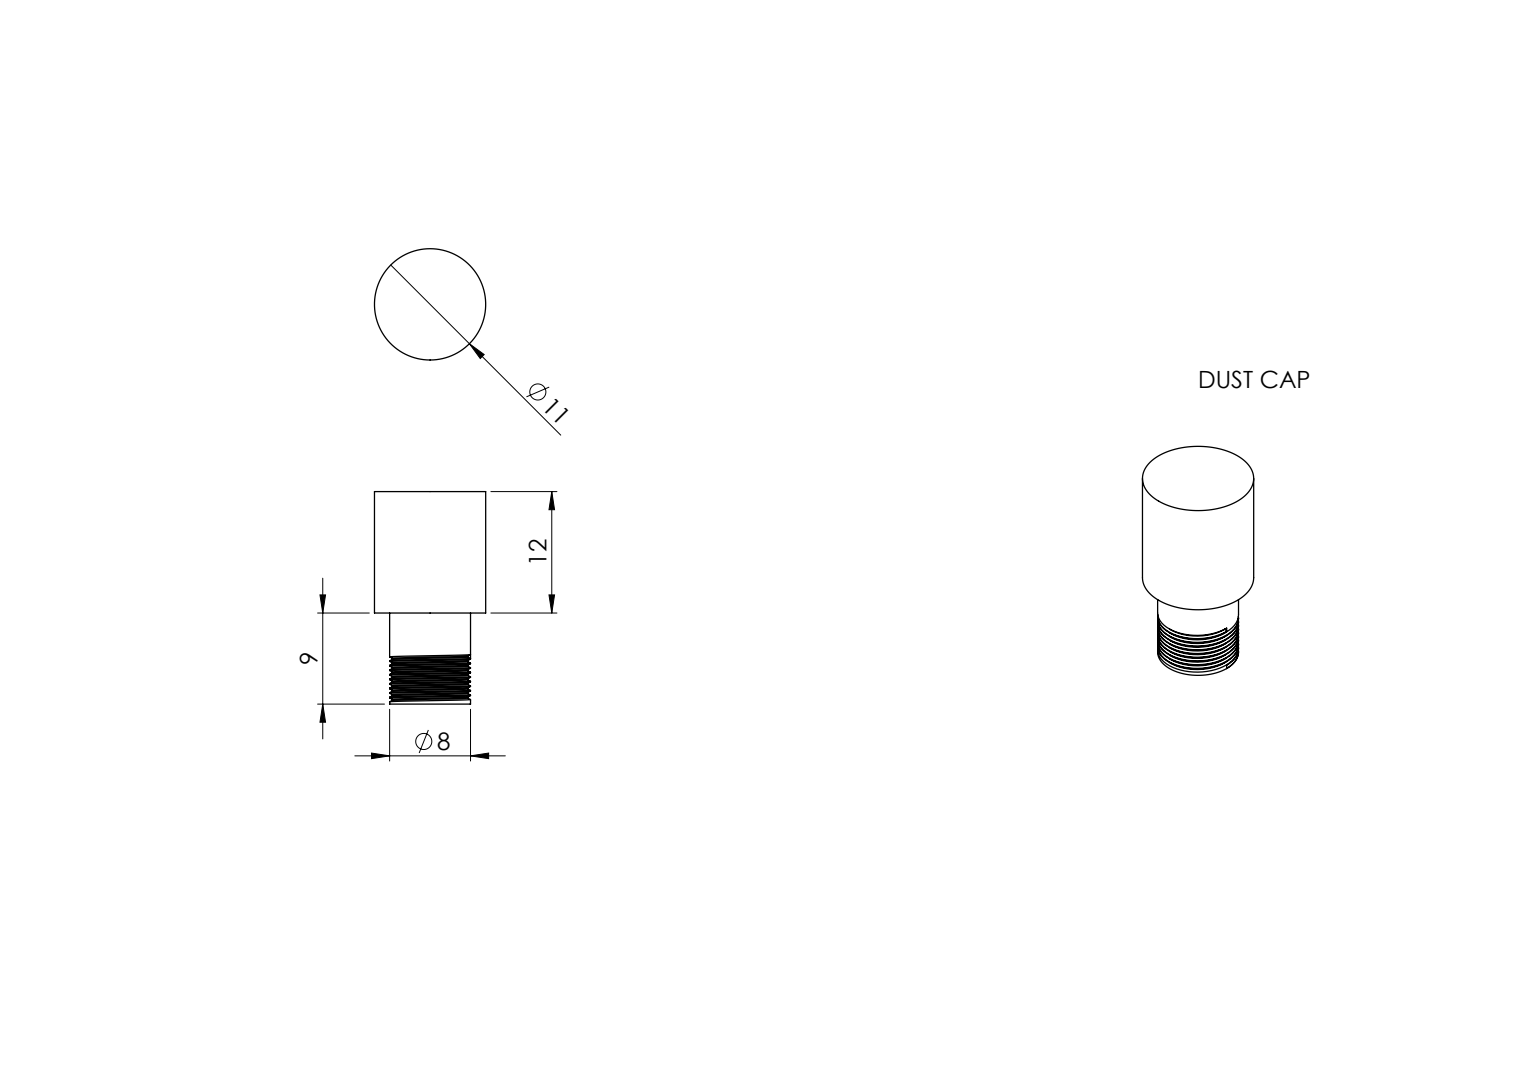
ISO-10303-21;
HEADER;
FILE_DESCRIPTION (('STEP AP214'),
    '1' );
FILE_NAME ('dust cap.step',
    '2026-10-26T12:50:16',
    ( '' ),
    ( '' ),
    'SwSTEP 2.0',
    'SolidWorks 2026',
    '' );
FILE_SCHEMA (( 'AUTOMOTIVE_DESIGN' ));
ENDSEC;

DATA;
#26=CARTESIAN_POINT ( 'NONE',  ( 3.959305671612554781E-15, 40.00000000000000000, 12.99999999999999289 ) ) ;
#57=CARTESIAN_POINT ( 'NONE',  ( 1.071796769724492338, 29.80134618820330417, 12.99999999999999467 ) ) ;
#68=CARTESIAN_POINT ( 'NONE',  ( -3.756430356249996994, 26.26562499938548711, 8.999999999999992895 ) ) ;
#90=CARTESIAN_POINT ( 'NONE',  ( 4.000000000000003553, 27.19374999877096855, 8.999999999999992895 ) ) ;
#94=CARTESIAN_POINT ( 'NONE',  ( 3.756430356250002323, 29.26562499938548356, 11.16877607737301403 ) ) ;
#120=CARTESIAN_POINT ( 'NONE',  ( 3.756430356250002323, 27.01562499938548356, 11.16877607737301226 ) ) ;
#140=VECTOR ( 'NONE', #15561, 1000.000000000000000 ) ;
#148=CARTESIAN_POINT ( 'NONE',  ( -3.756430356249997438, 26.30312499938548854, 11.16877607737301048 ) ) ;
#181=( BOUNDED_CURVE ( )  B_SPLINE_CURVE ( 2, ( #6217, #22433, #20464, #14467, #6482, #24270, #342, #4511, #8455 ),
 .UNSPECIFIED., .F., .T. ) 
 B_SPLINE_CURVE_WITH_KNOTS ( ( 3, 2, 2, 2, 3 ),
 ( 0.02500000000000000139, 0.03333333333333333287, 0.05000000000000000278, 0.06666666666666666574, 0.07500000000000001110 ),
 .UNSPECIFIED. ) 
 CURVE ( )  GEOMETRIC_REPRESENTATION_ITEM ( )  RATIONAL_B_SPLINE_CURVE ( ( 0.9330127018922194093, 0.9330127018922194093, 1.000000000000000000, 0.8660254037844387076, 1.000000000000000000, 0.8660254037844387076, 1.000000000000000000, 0.9330127018922191873, 0.9330127018922192983 ) ) 
 REPRESENTATION_ITEM ( '' )  );
#195=CARTESIAN_POINT ( 'NONE',  ( -3.756430356249997882, 27.20312499938548001, 11.16877607737301226 ) ) ;
#214=CARTESIAN_POINT ( 'NONE',  ( -1.999999999999995781, 28.69374999877096855, 5.535898384862237620 ) ) ;
#218=CARTESIAN_POINT ( 'NONE',  ( 3.756430356250002323, 27.46562499938548640, 11.16877607737301403 ) ) ;
#220=CARTESIAN_POINT ( 'NONE',  ( -3.999999999999997335, 27.90624999877097068, 11.30940107675849404 ) ) ;
#221=ORIENTED_EDGE ( 'NONE', *, *, #3705, .F. ) ;
#222=ORIENTED_EDGE ( 'NONE', *, *, #22140, .F. ) ;
#243=CARTESIAN_POINT ( 'NONE',  ( 3.756430356250003655, 29.75312499938548783, 8.999999999999992895 ) ) ;
#262=CARTESIAN_POINT ( 'NONE',  ( -3.999999999999997335, 27.00624999877096855, 11.30940107675849404 ) ) ;
#263=CARTESIAN_POINT ( 'NONE',  ( 3.834746474454188013E-15, 26.40624999877096357, 4.999999999999992006 ) ) ;
#269=LINE ( 'NONE', #15826, #13033 ) ;
#270=ADVANCED_FACE ( 'NONE', ( #14589 ), #20734, .T. ) ;
#271=CARTESIAN_POINT ( 'NONE',  ( -3.756430356249996994, 25.81562499938548427, 8.999999999999992895 ) ) ;
#287=ORIENTED_EDGE ( 'NONE', *, *, #24315, .F. ) ;
#291=CARTESIAN_POINT ( 'NONE',  ( 2.620986760973688460E-15, 29.38749999999999929, 13.61880215351699874 ) ) ;
#300=EDGE_CURVE ( 'NONE', #5668, #20971, #6231, .T. ) ;
#318=CARTESIAN_POINT ( 'NONE',  ( 2.672651547586948120E-15, 28.17812499938548143, 13.33755215474602984 ) ) ;
#334=CARTESIAN_POINT ( 'NONE',  ( -1.999999999999998224, 26.59374999877096712, 12.46410161513774639 ) ) ;
#342=CARTESIAN_POINT ( 'NONE',  ( -1.999999999999998224, 25.69374999877097210, 12.46410161513774639 ) ) ;
#367=CARTESIAN_POINT ( 'NONE',  ( -1.878215178124995832, 26.19062499938548427, 5.746835883940462963 ) ) ;
#378=( BOUNDED_SURFACE ( )  B_SPLINE_SURFACE ( 1, 2, ( 
 ( #13327, #4838, #19341, #20924, #22880, #1434, #9406, #21174, #3135, #17002, #12814, #4962, #7189, #20786, #15037, #25350, #2867, #13081, #11220, #6925, #23017, #1299, #25102, #18831, #16884, #24849, #12943, #3008, #5102, #19080, #21056, #1160, #9139, #17891, #17645, #21682, #17504, #1943, #3518, #25864, #15939, #3767, #9522, #1554, #21822, #11746, #11489, #120, #9906, #11875, #9662, #25615, #7952, #19726, #15556, #25482, #1823, #13976, #7819, #7568, #11990, #23525, #23911, #18034, #23770, #5859, #13843, #1686, #8091, #3904, #15800, #5992, #19842, #7699, #19964, #5609, #21945, #4023, #2068, #10036, #9787, #23392, #17767, #13589, #15680, #5476, #25736, #5725, #13471, #21437, #19462, #21556, #3636, #11608, #19582, #23648, #13706, #4676, #10672, #22594, #20627, #12655, #2710, #10549, #12262, #18662, #18165, #2327, #20231, #18548, #10286, #12513, #6115, #4291, #16325, #4150, #2586, #22063, #16070, #16187, #243 ),
 ( #505, #8213, #8475, #749, #24153, #16461, #2208, #24033, #14098, #10408, #6244, #16579, #12128, #20104, #10167, #6623, #24538, #22329, #24294, #4411, #14234, #22204, #6379, #18279, #24423, #2447, #6500, #14485, #367, #18407, #8337, #14369, #12385, #20489, #14613, #22452, #20351, #4533, #630, #8597, #3101, #21023, #1013, #4808, #24934, #3347, #8990, #10801, #2833, #13173, #6764, #9102, #21142, #19168, #11184, #25065, #3214, #24678, #11067, #13290, #19045, #17092, #881, #7284, #12783, #20755, #14750, #16967, #18793, #22728, #8864, #1261, #21266, #1128, #16850, #25206, #24814, #7153, #4924, #14875, #23112, #9246, #15143, #15261, #17234, #15000, #12908, #19305, #23229, #5312, #6892, #5194, #11323, #8718, #16705, #2972, #13044, #22850, #20884, #10939, #18930, #7013, #22979, #5065, #21911, #5441, #15767, #13673, #23733, #21644, #9623, #15523, #23491, #23352, #3727, #7401, #9756, #17735, #19429, #3604, #1402 ) ),
 .UNSPECIFIED., .F., .F., .F. ) 
 B_SPLINE_SURFACE_WITH_KNOTS ( ( 2, 2 ),
 ( 3, 2, 2, 2, 2, 2, 2, 2, 2, 2, 2, 2, 2, 2, 2, 2, 2, 2, 2, 2, 2, 2, 2, 2, 2, 2, 2, 2, 2, 2, 2, 2, 2, 2, 2, 2, 2, 2, 2, 2, 2, 2, 2, 2, 2, 2, 2, 2, 2, 2, 2, 2, 2, 2, 2, 2, 2, 2, 2, 2, 3 ),
 ( 0.000000000000000000, 1.000000000000000000 ),
 ( 0.000000000000000000, 0.01666666666666666644, 0.03333333333333333287, 0.05000000000000000278, 0.06666666666666666574, 0.08333333333333332871, 0.1000000000000000056, 0.1166666666666666685, 0.1333333333333333315, 0.1499999999999999944, 0.1666666666666666574, 0.1833333333333333204, 0.2000000000000000111, 0.2166666666666666741, 0.2333333333333333370, 0.2500000000000000000, 0.2666666666666666630, 0.2833333333333333259, 0.2999999999999999889, 0.3166666666666666519, 0.3333333333333333148, 0.3499999999999999778, 0.3666666666666666408, 0.3833333333333333592, 0.4000000000000000222, 0.4166666666666666852, 0.4333333333333333481, 0.4500000000000000111, 0.4666666666666666741, 0.4833333333333333370, 0.5000000000000000000, 0.5166666666666667185, 0.5333333333333333259, 0.5500000000000000444, 0.5666666666666666519, 0.5833333333333333703, 0.5999999999999999778, 0.6166666666666666963, 0.6333333333333333037, 0.6500000000000000222, 0.6666666666666666297, 0.6833333333333333481, 0.6999999999999999556, 0.7166666666666666741, 0.7333333333333332815, 0.7500000000000000000, 0.7666666666666667185, 0.7833333333333333259, 0.8000000000000000444, 0.8166666666666666519, 0.8333333333333333703, 0.8499999999999999778, 0.8666666666666666963, 0.8833333333333333037, 0.9000000000000000222, 0.9166666666666666297, 0.9333333333333333481, 0.9499999999999999556, 0.9666666666666666741, 0.9833333333333332815, 1.000000000000000000 ),
 .UNSPECIFIED. ) 
 GEOMETRIC_REPRESENTATION_ITEM ( )  RATIONAL_B_SPLINE_SURFACE ( (
 ( 1.000000000000000000, 0.8660254037844387076, 1.000000000000000000, 0.8660254037844387076, 1.000000000000000000, 0.8660254037844387076, 1.000000000000000000, 0.8660254037844387076, 1.000000000000000000, 0.8660254037844387076, 1.000000000000000000, 0.8660254037844387076, 1.000000000000000000, 0.8660254037844387076, 1.000000000000000000, 0.8660254037844387076, 1.000000000000000000, 0.8660254037844387076, 1.000000000000000000, 0.8660254037844387076, 1.000000000000000000, 0.8660254037844387076, 1.000000000000000000, 0.8660254037844387076, 1.000000000000000000, 0.8660254037844387076, 1.000000000000000000, 0.8660254037844387076, 1.000000000000000000, 0.8660254037844387076, 1.000000000000000000, 0.8660254037844387076, 1.000000000000000000, 0.8660254037844387076, 1.000000000000000000, 0.8660254037844387076, 1.000000000000000000, 0.8660254037844387076, 1.000000000000000000, 0.8660254037844387076, 1.000000000000000000, 0.8660254037844387076, 1.000000000000000000, 0.8660254037844387076, 1.000000000000000000, 0.8660254037844387076, 1.000000000000000000, 0.8660254037844387076, 1.000000000000000000, 0.8660254037844387076, 1.000000000000000000, 0.8660254037844387076, 1.000000000000000000, 0.8660254037844387076, 1.000000000000000000, 0.8660254037844387076, 1.000000000000000000, 0.8660254037844387076, 1.000000000000000000, 0.8660254037844387076, 1.000000000000000000, 0.8660254037844387076, 1.000000000000000000, 0.8660254037844387076, 1.000000000000000000, 0.8660254037844387076, 1.000000000000000000, 0.8660254037844387076, 1.000000000000000000, 0.8660254037844387076, 1.000000000000000000, 0.8660254037844387076, 1.000000000000000000, 0.8660254037844387076, 1.000000000000000000, 0.8660254037844387076, 1.000000000000000000, 0.8660254037844387076, 1.000000000000000000, 0.8660254037844387076, 1.000000000000000000, 0.8660254037844387076, 1.000000000000000000, 0.8660254037844387076, 1.000000000000000000, 0.8660254037844387076, 1.000000000000000000, 0.8660254037844387076, 1.000000000000000000, 0.8660254037844387076, 1.000000000000000000, 0.8660254037844387076, 1.000000000000000000, 0.8660254037844387076, 1.000000000000000000, 0.8660254037844387076, 1.000000000000000000, 0.8660254037844387076, 1.000000000000000000, 0.8660254037844387076, 1.000000000000000000, 0.8660254037844387076, 1.000000000000000000, 0.8660254037844387076, 1.000000000000000000, 0.8660254037844387076, 1.000000000000000000, 0.8660254037844387076, 1.000000000000000000, 0.8660254037844387076, 1.000000000000000000, 0.8660254037844387076, 1.000000000000000000, 0.8660254037844387076, 1.000000000000000000, 0.8660254037844387076, 1.000000000000000000, 0.8660254037844387076, 1.000000000000000000, 0.8660254037844387076, 1.000000000000000000),
 ( 1.000000000000000000, 0.8660254037844387076, 1.000000000000000000, 0.8660254037844387076, 1.000000000000000000, 0.8660254037844387076, 1.000000000000000000, 0.8660254037844387076, 1.000000000000000000, 0.8660254037844387076, 1.000000000000000000, 0.8660254037844387076, 1.000000000000000000, 0.8660254037844387076, 1.000000000000000000, 0.8660254037844387076, 1.000000000000000000, 0.8660254037844387076, 1.000000000000000000, 0.8660254037844387076, 1.000000000000000000, 0.8660254037844387076, 1.000000000000000000, 0.8660254037844387076, 1.000000000000000000, 0.8660254037844387076, 1.000000000000000000, 0.8660254037844387076, 1.000000000000000000, 0.8660254037844387076, 1.000000000000000000, 0.8660254037844387076, 1.000000000000000000, 0.8660254037844387076, 1.000000000000000000, 0.8660254037844387076, 1.000000000000000000, 0.8660254037844387076, 1.000000000000000000, 0.8660254037844387076, 1.000000000000000000, 0.8660254037844387076, 1.000000000000000000, 0.8660254037844387076, 1.000000000000000000, 0.8660254037844387076, 1.000000000000000000, 0.8660254037844387076, 1.000000000000000000, 0.8660254037844387076, 1.000000000000000000, 0.8660254037844387076, 1.000000000000000000, 0.8660254037844387076, 1.000000000000000000, 0.8660254037844387076, 1.000000000000000000, 0.8660254037844387076, 1.000000000000000000, 0.8660254037844387076, 1.000000000000000000, 0.8660254037844387076, 1.000000000000000000, 0.8660254037844387076, 1.000000000000000000, 0.8660254037844387076, 1.000000000000000000, 0.8660254037844387076, 1.000000000000000000, 0.8660254037844387076, 1.000000000000000000, 0.8660254037844387076, 1.000000000000000000, 0.8660254037844387076, 1.000000000000000000, 0.8660254037844387076, 1.000000000000000000, 0.8660254037844387076, 1.000000000000000000, 0.8660254037844387076, 1.000000000000000000, 0.8660254037844387076, 1.000000000000000000, 0.8660254037844387076, 1.000000000000000000, 0.8660254037844387076, 1.000000000000000000, 0.8660254037844387076, 1.000000000000000000, 0.8660254037844387076, 1.000000000000000000, 0.8660254037844387076, 1.000000000000000000, 0.8660254037844387076, 1.000000000000000000, 0.8660254037844387076, 1.000000000000000000, 0.8660254037844387076, 1.000000000000000000, 0.8660254037844387076, 1.000000000000000000, 0.8660254037844387076, 1.000000000000000000, 0.8660254037844387076, 1.000000000000000000, 0.8660254037844387076, 1.000000000000000000, 0.8660254037844387076, 1.000000000000000000, 0.8660254037844387076, 1.000000000000000000, 0.8660254037844387076, 1.000000000000000000, 0.8660254037844387076, 1.000000000000000000, 0.8660254037844387076, 1.000000000000000000, 0.8660254037844387076, 1.000000000000000000, 0.8660254037844387076, 1.000000000000000000) ) ) 
 REPRESENTATION_ITEM ( '' )  SURFACE ( )  );
#381=EDGE_LOOP ( 'NONE', ( #3819, #17426, #15116, #9054 ) ) ;
#397=CARTESIAN_POINT ( 'NONE',  ( -3.756430356249996105, 25.77812499938548285, 6.831223922626973533 ) ) ;
#408=VERTEX_POINT ( 'NONE', #21244 ) ;
#457=CARTESIAN_POINT ( 'NONE',  ( 2.672651547586948120E-15, 27.27812499938548285, 13.33755215474602984 ) ) ;
#473=CARTESIAN_POINT ( 'NONE',  ( 3.369928719974892281E-15, 25.11250000000000426, 4.999999999999992006 ) ) ;
#477=CARTESIAN_POINT ( 'NONE',  ( -3.756430356249995661, 25.44062499938548427, 6.831223922626973533 ) ) ;
#481=ORIENTED_EDGE ( 'NONE', *, *, #22170, .T. ) ;
#505=CARTESIAN_POINT ( 'NONE',  ( 3.756430356250003655, 25.14062499938548356, 8.999999999999992895 ) ) ;
#535=CARTESIAN_POINT ( 'NONE',  ( -1.878215178124998497, 26.34062499938548285, 12.25316411605951927 ) ) ;
#581=CARTESIAN_POINT ( 'NONE',  ( 1.071796769724494336, 25.09240381056766367, 4.999999999999992895 ) ) ;
#591=CARTESIAN_POINT ( 'NONE',  ( -1.878215178124995832, 27.54062499938548214, 5.746835883940462963 ) ) ;
#597=CARTESIAN_POINT ( 'NONE',  ( 3.369928719974892281E-15, 25.11250000000000426, 4.999999999999992006 ) ) ;
#607=CARTESIAN_POINT ( 'NONE',  ( 3.735045420075836212E-15, 26.26562499938548356, 4.662447845253954171 ) ) ;
#613=( BOUNDED_CURVE ( )  B_SPLINE_CURVE ( 2, ( #5584, #19696, #5450, #11464, #9881 ),
 .UNSPECIFIED., .F., .F. ) 
 B_SPLINE_CURVE_WITH_KNOTS ( ( 3, 2, 3 ),
 ( 0.9749999999999999778, 0.9833333333333332815, 1.000000000000000000 ),
 .UNSPECIFIED. ) 
 CURVE ( )  GEOMETRIC_REPRESENTATION_ITEM ( )  RATIONAL_B_SPLINE_CURVE ( ( 0.9330127018922194093, 0.9330127018922194093, 1.000000000000000000, 0.8660254037844387076, 1.000000000000000000 ) ) 
 REPRESENTATION_ITEM ( '' )  );
#630=CARTESIAN_POINT ( 'NONE',  ( 1.878215178125004048, 26.56562499938548427, 5.746835883940462963 ) ) ;
#632=EDGE_LOOP ( 'NONE', ( #6319, #11612, #8419, #5612 ) ) ;
#657=CARTESIAN_POINT ( 'NONE',  ( 3.756430356250003211, 28.32812499938548356, 6.831223922626973533 ) ) ;
#667=DIRECTION ( 'NONE',  ( 0.000000000000000000, -1.000000000000000000, 0.000000000000000000 ) ) ;
#671=EDGE_LOOP ( 'NONE', ( #19623, #22738 ) ) ;
#683=DIRECTION ( 'NONE',  ( -0.000000000000000000, -1.000000000000000000, -0.000000000000000000 ) ) ;
#706=CARTESIAN_POINT ( 'NONE',  ( 1.071796769724494558, 28.63615380933863364, 4.999999999999992895 ) ) ;
#708=CARTESIAN_POINT ( 'NONE',  ( -3.756430356249996994, 28.51562499938548356, 8.999999999999992895 ) ) ;
#714=EDGE_CURVE ( 'NONE', #10206, #12794, #12708, .T. ) ;
#721=CARTESIAN_POINT ( 'NONE',  ( -1.057460391440397258E-14, 28.71250000000000213, 4.999999999999992006 ) ) ;
#723=CARTESIAN_POINT ( 'NONE',  ( 3.756430356250003655, 26.15312499938548640, 8.999999999999992895 ) ) ;
#728=CARTESIAN_POINT ( 'NONE',  ( 3.756430356250003655, 29.75312499938548783, 8.999999999999992895 ) ) ;
#729=DIRECTION ( 'NONE',  ( 0.000000000000000000, 0.000000000000000000, -1.000000000000000000 ) ) ;
#749=CARTESIAN_POINT ( 'NONE',  ( 3.735045420075836212E-15, 25.25312499938548783, 4.662447845253954171 ) ) ;
#775=CARTESIAN_POINT ( 'NONE',  ( -3.756430356249996994, 29.41562499938548569, 8.999999999999992895 ) ) ;
#803=CARTESIAN_POINT ( 'NONE',  ( 1.859271017917182139E-15, 28.48749999999999716, 12.99999999999999289 ) ) ;
#820=AXIS2_PLACEMENT_3D ( 'NONE', #8589, #18784, #24666 ) ;
#830=ORIENTED_EDGE ( 'NONE', *, *, #3925, .F. ) ;
#832=CARTESIAN_POINT ( 'NONE',  ( 1.878215178125000939, 29.11562499938548498, 12.25316411605952283 ) ) ;
#841=EDGE_CURVE ( 'NONE', #11726, #2271, #16535, .T. ) ;
#851=CARTESIAN_POINT ( 'NONE',  ( -3.999999999999996003, 29.18124999877096926, 6.690598923241487306 ) ) ;
#881=CARTESIAN_POINT ( 'NONE',  ( 1.878215178125004048, 27.46562499938548640, 5.746835883940462963 ) ) ;
#897=ORIENTED_EDGE ( 'NONE', *, *, #8841, .F. ) ;
#910=( BOUNDED_CURVE ( )  B_SPLINE_CURVE ( 2, ( #13594, #7704, #19208, #23776, #5349, #9288, #7824, #17391, #1829 ),
 .UNSPECIFIED., .F., .F. ) 
 B_SPLINE_CURVE_WITH_KNOTS ( ( 3, 2, 2, 2, 3 ),
 ( 0.4750000000000000333, 0.4833333333333333370, 0.5000000000000000000, 0.5166666666666667185, 0.5250000000000000222 ),
 .UNSPECIFIED. ) 
 CURVE ( )  GEOMETRIC_REPRESENTATION_ITEM ( )  RATIONAL_B_SPLINE_CURVE ( ( 0.9330127018922194093, 0.9330127018922196314, 1.000000000000000000, 0.8660254037844387076, 1.000000000000000000, 0.8660254037844387076, 1.000000000000000000, 0.9330127018922194093, 0.9330127018922194093 ) ) 
 REPRESENTATION_ITEM ( '' )  );
#914=CARTESIAN_POINT ( 'NONE',  ( 3.756430356250002323, 29.60312499938548569, 11.16877607737301403 ) ) ;
#966=ORIENTED_EDGE ( 'NONE', *, *, #11818, .F. ) ;
#971=CARTESIAN_POINT ( 'NONE',  ( -1.878215178124998497, 29.04062499938548569, 12.25316411605951927 ) ) ;
#986=CARTESIAN_POINT ( 'NONE',  ( -1.999999999999995781, 29.14374999877096784, 5.535898384862237620 ) ) ;
#1005=ADVANCED_FACE ( 'NONE', ( #19741 ), #11764, .T. ) ;
#1013=CARTESIAN_POINT ( 'NONE',  ( -3.756430356249996994, 26.71562499938548285, 8.999999999999992895 ) ) ;
#1042=CARTESIAN_POINT ( 'NONE',  ( 1.878215178125004048, 29.26562499938548356, 5.746835883940462963 ) ) ;
#1044=LINE ( 'NONE', #17127, #12204 ) ;
#1048=CARTESIAN_POINT ( 'NONE',  ( 3.834746474454188013E-15, 27.75624999877096855, 4.999999999999992006 ) ) ;
#1068=EDGE_CURVE ( 'NONE', #1940, #9674, #15367, .T. ) ;
#1085=ORIENTED_EDGE ( 'NONE', *, *, #12027, .F. ) ;
#1089=CARTESIAN_POINT ( 'NONE',  ( 4.000000000000003553, 25.00000000000000000, 8.999999999999992895 ) ) ;
#1104=CARTESIAN_POINT ( 'NONE',  ( 3.756430356250003655, 27.50312499938548427, 8.999999999999992895 ) ) ;
#1110=CARTESIAN_POINT ( 'NONE',  ( 1.071796769724492338, 26.20134618820330275, 12.99999999999999467 ) ) ;
#1128=CARTESIAN_POINT ( 'NONE',  ( 3.756430356250004099, 27.87812499938548427, 6.831223922626973533 ) ) ;
#1135=CARTESIAN_POINT ( 'NONE',  ( -3.999999999999995559, 28.78750000000000142, 6.690598923241487306 ) ) ;
#1140=CARTESIAN_POINT ( 'NONE',  ( 1.878215178125000939, 26.07812499938548356, 12.25316411605952283 ) ) ;
#1154=CARTESIAN_POINT ( 'NONE',  ( 2.672651547586948120E-15, 28.62812499938548783, 13.33755215474603162 ) ) ;
#1160=CARTESIAN_POINT ( 'NONE',  ( -3.756430356249997882, 26.41562499938548569, 11.16877607737301226 ) ) ;
#1161=CARTESIAN_POINT ( 'NONE',  ( 4.000000000000003553, 27.68124999877096926, 6.690598923241489970 ) ) ;
#1168=VERTEX_POINT ( 'NONE', #8701 ) ;
#1172=EDGE_LOOP ( 'NONE', ( #1838, #14310, #24792, #24076 ) ) ;
#1177=DIRECTION ( 'NONE',  ( -0.000000000000000000, -1.000000000000000000, -0.000000000000000000 ) ) ;
#1214=CARTESIAN_POINT ( 'NONE',  ( -1.878215178124998497, 28.59062499938548285, 12.25316411605951927 ) ) ;
#1219=CARTESIAN_POINT ( 'NONE',  ( -3.999999999999996447, 26.57500000000000284, 8.999999999999992895 ) ) ;
#1233=CARTESIAN_POINT ( 'NONE',  ( -3.756430356249996994, 27.27812499938548640, 8.999999999999992895 ) ) ;
#1261=CARTESIAN_POINT ( 'NONE',  ( 3.756430356250002323, 27.80312499938548143, 11.16877607737301226 ) ) ;
#1273=CARTESIAN_POINT ( 'NONE',  ( -3.756430356249997438, 25.96562499938548640, 11.16877607737301048 ) ) ;
#1299=CARTESIAN_POINT ( 'NONE',  ( 2.672651547586948120E-15, 26.04062499938548925, 13.33755215474602984 ) ) ;
#1300=CARTESIAN_POINT ( 'NONE',  ( 2.000000000000003997, 27.71874999877097068, 5.535898384862238508 ) ) ;
#1305=VERTEX_POINT ( 'NONE', #5426 ) ;
#1326=ADVANCED_FACE ( 'NONE', ( #13414 ), #3053, .T. ) ;
#1356=CARTESIAN_POINT ( 'NONE',  ( -3.999999999999997335, 27.96250000000000213, 11.30940107675849404 ) ) ;
#1359=CARTESIAN_POINT ( 'NONE',  ( -3.137519842735244810E-15, 26.46249999999999858, 4.999999999999991118 ) ) ;
#1360=PRODUCT_DEFINITION ( 'UNKNOWN', '', #16061, #7043 ) ;
#1365=EDGE_CURVE ( 'NONE', #21478, #1940, #2376, .T. ) ;
#1376=CARTESIAN_POINT ( 'NONE',  ( 1.878215178125000939, 27.42812499938548498, 12.25316411605952283 ) ) ;
#1395=FACE_OUTER_BOUND ( 'NONE', #2684, .T. ) ;
#1402=CARTESIAN_POINT ( 'NONE',  ( 3.756430356250003655, 29.64062499938548356, 8.999999999999992895 ) ) ;
#1407=CARTESIAN_POINT ( 'NONE',  ( 2.000000000000000888, 25.76874999877096784, 12.46410161513774817 ) ) ;
#1412=CARTESIAN_POINT ( 'NONE',  ( 1.878215178125000939, 26.97812499938548569, 12.25316411605952283 ) ) ;
#1434=CARTESIAN_POINT ( 'NONE',  ( -3.756430356249995661, 25.44062499938548427, 6.831223922626973533 ) ) ;
#1472=ORIENTED_EDGE ( 'NONE', *, *, #300, .F. ) ;
#1477=CARTESIAN_POINT ( 'NONE',  ( 4.000000000000003553, 26.83749999999999503, 6.690598923241489970 ) ) ;
#1478=ORIENTED_EDGE ( 'NONE', *, *, #8035, .F. ) ;
#1480=CARTESIAN_POINT ( 'NONE',  ( 3.752267015613588906E-15, 28.26250000000000284, 4.381197846482986158 ) ) ;
#1481=CARTESIAN_POINT ( 'NONE',  ( 3.469446951953614189E-15, 46.00000000000000000, 8.999999999999992895 ) ) ;
#1482=CARTESIAN_POINT ( 'NONE',  ( -3.999999999999995559, 26.53750000000000142, 6.690598923241487306 ) ) ;
#1497=CARTESIAN_POINT ( 'NONE',  ( -1.878215178124995832, 28.55312499938548498, 5.746835883940462963 ) ) ;
#1506=CARTESIAN_POINT ( 'NONE',  ( 1.878215178125004048, 25.66562499938548569, 5.746835883940462963 ) ) ;
#1525=CARTESIAN_POINT ( 'NONE',  ( -3.999999999999996003, 25.58124999877097139, 6.690598923241487306 ) ) ;
#1527=FACE_OUTER_BOUND ( 'NONE', #671, .T. ) ;
#1529=CARTESIAN_POINT ( 'NONE',  ( 3.756430356250003211, 26.19062499938548783, 6.831223922626973533 ) ) ;
#1531=ORIENTED_EDGE ( 'NONE', *, *, #3720, .T. ) ;
#1554=CARTESIAN_POINT ( 'NONE',  ( -3.756430356249997882, 26.86562499938548498, 11.16877607737301226 ) ) ;
#1559=DIRECTION ( 'NONE',  ( 0.000000000000000000, 1.000000000000000000, 0.000000000000000000 ) ) ;
#1603=CARTESIAN_POINT ( 'NONE',  ( 4.000000000000003553, 26.38750000000000284, 6.690598923241489970 ) ) ;
#1617=AXIS2_PLACEMENT_3D ( 'NONE', #19728, #19843, #5727 ) ;
#1621=CARTESIAN_POINT ( 'NONE',  ( 3.756430356250004099, 27.09062499938548285, 6.831223922626973533 ) ) ;
#1630=CARTESIAN_POINT ( 'NONE',  ( -3.756430356249996994, 25.36562499938548498, 8.999999999999992895 ) ) ;
#1640=CARTESIAN_POINT ( 'NONE',  ( -3.999999999999997335, 27.51250000000000284, 11.30940107675849404 ) ) ;
#1654=CARTESIAN_POINT ( 'NONE',  ( -3.999999999999996447, 26.06874999877096855, 8.999999999999992895 ) ) ;
#1658=CARTESIAN_POINT ( 'NONE',  ( -3.756430356249996105, 26.34062499938548285, 6.831223922626973533 ) ) ;
#1665=VERTEX_POINT ( 'NONE', #2239 ) ;
#1686=CARTESIAN_POINT ( 'NONE',  ( -3.756430356249997882, 27.76562499938549067, 11.16877607737301226 ) ) ;
#1702=ORIENTED_EDGE ( 'NONE', *, *, #22026, .T. ) ;
#1718=FACE_OUTER_BOUND ( 'NONE', #4223, .T. ) ;
#1720=LINE ( 'NONE', #18068, #3840 ) ;
#1734=LINE ( 'NONE', #26, #23734 ) ;
#1741=CIRCLE ( 'NONE', #5077, 5.500000000000000000 ) ;
#1742=ORIENTED_EDGE ( 'NONE', *, *, #11468, .F. ) ;
#1743=CARTESIAN_POINT ( 'NONE',  ( 2.000000000000000888, 27.62500000000000000, 12.46410161513774817 ) ) ;
#1745=VECTOR ( 'NONE', #14065, 1000.000000000000000 ) ;
#1750=( BOUNDED_CURVE ( )  B_SPLINE_CURVE ( 2, ( #23869, #8175, #5954, #17730, #23996, #1640, #19806, #25699, #18130 ),
 .UNSPECIFIED., .F., .F. ) 
 B_SPLINE_CURVE_WITH_KNOTS ( ( 3, 2, 2, 2, 3 ),
 ( 0.5250000000000000222, 0.5333333333333333259, 0.5500000000000000444, 0.5666666666666666519, 0.5750000000000000666 ),
 .UNSPECIFIED. ) 
 CURVE ( )  GEOMETRIC_REPRESENTATION_ITEM ( )  RATIONAL_B_SPLINE_CURVE ( ( 0.9330127018922194093, 0.9330127018922194093, 1.000000000000000000, 0.8660254037844387076, 1.000000000000000000, 0.8660254037844387076, 1.000000000000000000, 0.9330127018922189652, 0.9330127018922194093 ) ) 
 REPRESENTATION_ITEM ( '' )  );
#1752=CYLINDRICAL_SURFACE ( 'NONE', #20479, 4.000000000000000000 ) ;
#1767=CARTESIAN_POINT ( 'NONE',  ( 3.756430356250004099, 29.34062499938548640, 6.831223922626973533 ) ) ;
#1793=CARTESIAN_POINT ( 'NONE',  ( -1.999999999999995781, 25.99374999877096926, 5.535898384862237620 ) ) ;
#1797=CARTESIAN_POINT ( 'NONE',  ( 2.672651547586948120E-15, 27.84062499938548640, 13.33755215474603162 ) ) ;
#1823=CARTESIAN_POINT ( 'NONE',  ( -1.878215178124998497, 27.35312499938548569, 12.25316411605951927 ) ) ;
#1829=CARTESIAN_POINT ( 'NONE',  ( 3.834746474454188013E-15, 27.36250000000000426, 4.999999999999992006 ) ) ;
#1838=ORIENTED_EDGE ( 'NONE', *, *, #4123, .F. ) ;
#1857=CARTESIAN_POINT ( 'NONE',  ( 1.626862140677534194E-14, 27.58750000000000213, 12.99999999999999289 ) ) ;
#1865=( BOUNDED_CURVE ( )  B_SPLINE_CURVE ( 2, ( #8288, #10502, #16271, #24241, #8427, #24382, #6458, #706, #14446 ),
 .UNSPECIFIED., .F., .F. ) 
 B_SPLINE_CURVE_WITH_KNOTS ( ( 3, 2, 2, 2, 3 ),
 ( 0.6750000000000000444, 0.6833333333333333481, 0.6999999999999999556, 0.7166666666666666741, 0.7249999999999999778 ),
 .UNSPECIFIED. ) 
 CURVE ( )  GEOMETRIC_REPRESENTATION_ITEM ( )  RATIONAL_B_SPLINE_CURVE ( ( 0.9330127018922194093, 0.9330127018922198534, 1.000000000000000000, 0.8660254037844387076, 1.000000000000000000, 0.8660254037844387076, 1.000000000000000000, 0.9330127018922194093, 0.9330127018922194093 ) ) 
 REPRESENTATION_ITEM ( '' )  );
#1869=CARTESIAN_POINT ( 'NONE',  ( 3.369928719974892281E-15, 25.50624999877096855, 4.999999999999992006 ) ) ;
#1872=CARTESIAN_POINT ( 'NONE',  ( 4.000000000000003553, 26.80000000000000071, 8.999999999999992895 ) ) ;
#1874=ADVANCED_FACE ( 'NONE', ( #24967 ), #378, .T. ) ;
#1907=EDGE_CURVE ( 'NONE', #10879, #16189, #17053, .T. ) ;
#1918=CARTESIAN_POINT ( 'NONE',  ( -1.999999999999998224, 28.39374999877096784, 12.46410161513774639 ) ) ;
#1922=CARTESIAN_POINT ( 'NONE',  ( 2.672651547586948120E-15, 28.74062499938548854, 13.33755215474603162 ) ) ;
#1940=VERTEX_POINT ( 'NONE', #13557 ) ;
#1943=CARTESIAN_POINT ( 'NONE',  ( 3.756430356250004099, 26.64062499938549067, 6.831223922626973533 ) ) ;
#1949=DIRECTION ( 'NONE',  ( -0.000000000000000000, -1.000000000000000000, -0.000000000000000000 ) ) ;
#1958=ADVANCED_FACE ( 'NONE', ( #21523 ), #11575, .T. ) ;
#1962=SURFACE_SIDE_STYLE ('',( #8501 ) ) ;
#1964=EDGE_CURVE ( 'NONE', #12794, #16109, #10013, .T. ) ;
#1986=CARTESIAN_POINT ( 'NONE',  ( 1.071796769724494336, 25.48615380933863150, 4.999999999999992895 ) ) ;
#1994=CARTESIAN_POINT ( 'NONE',  ( 3.834746474454188013E-15, 26.01249999999999574, 4.999999999999992006 ) ) ;
#2008=CARTESIAN_POINT ( 'NONE',  ( 2.672651547586948120E-15, 29.19062499938548783, 13.33755215474602984 ) ) ;
#2017=CARTESIAN_POINT ( 'NONE',  ( 3.756430356250003655, 26.04062499938548569, 8.999999999999992895 ) ) ;
#2024=CARTESIAN_POINT ( 'NONE',  ( 8.831537335106614961E-15, 27.13750000000000284, 12.99999999999999112 ) ) ;
#2039=CARTESIAN_POINT ( 'NONE',  ( 2.000000000000000888, 27.56874999877096855, 12.46410161513774817 ) ) ;
#2043=CARTESIAN_POINT ( 'NONE',  ( 3.756430356250003211, 27.99062499938548498, 6.831223922626973533 ) ) ;
#2057=AXIS2_PLACEMENT_3D ( 'NONE', #24683, #18412, #24817 ) ;
#2062=CARTESIAN_POINT ( 'NONE',  ( 1.071796769724494558, 25.54240381056766651, 4.999999999999992895 ) ) ;
#2068=CARTESIAN_POINT ( 'NONE',  ( -3.756430356249996994, 28.17812499938548498, 8.999999999999992895 ) ) ;
#2093=( NAMED_UNIT ( * ) SI_UNIT ( $, .STERADIAN. ) SOLID_ANGLE_UNIT ( ) );
#2097=CARTESIAN_POINT ( 'NONE',  ( 3.756430356250003211, 25.17812499938548498, 6.831223922626973533 ) ) ;
#2155=CARTESIAN_POINT ( 'NONE',  ( 1.878215178125004048, 26.56562499938548427, 5.746835883940462963 ) ) ;
#2176=CARTESIAN_POINT ( 'NONE',  ( -3.999999999999996447, 28.31874999877096855, 8.999999999999992895 ) ) ;
#2180=CARTESIAN_POINT ( 'NONE',  ( 1.878215178125000939, 28.32812499938548711, 12.25316411605952283 ) ) ;
#2193=CIRCLE ( 'NONE', #16817, 5.500000000000000000 ) ;
#2208=CARTESIAN_POINT ( 'NONE',  ( -3.756430356249996994, 25.36562499938548498, 8.999999999999992895 ) ) ;
#2209=AXIS2_PLACEMENT_3D ( 'NONE', #23562, #4189, #23679 ) ;
#2234=CARTESIAN_POINT ( 'NONE',  ( -3.756430356249996105, 25.32812499938548356, 6.831223922626973533 ) ) ;
#2239=CARTESIAN_POINT ( 'NONE',  ( 3.834746474454188013E-15, 27.36250000000000071, 4.999999999999992006 ) ) ;
#2255=CARTESIAN_POINT ( 'NONE',  ( 2.620986760973688460E-15, 28.93750000000000000, 13.61880215351699874 ) ) ;
#2271=VERTEX_POINT ( 'NONE', #18756 ) ;
#2283=CARTESIAN_POINT ( 'NONE',  ( -1.878215178124998497, 28.14062499938548356, 12.25316411605951927 ) ) ;
#2300=CARTESIAN_POINT ( 'NONE',  ( 2.000000000000000888, 26.66874999877096641, 12.46410161513774817 ) ) ;
#2309=CARTESIAN_POINT ( 'NONE',  ( 4.000000000000003553, 29.89374999877096784, 8.999999999999992895 ) ) ;
#2327=CARTESIAN_POINT ( 'NONE',  ( 3.756430356250002323, 29.26562499938548356, 11.16877607737301226 ) ) ;
#2338=ORIENTED_EDGE ( 'NONE', *, *, #8279, .F. ) ;
#2345=EDGE_CURVE ( 'NONE', #22108, #19820, #19079, .T. ) ;
#2350=SURFACE_STYLE_USAGE ( .BOTH. , #1962 ) ;
#2354=CARTESIAN_POINT ( 'NONE',  ( -3.756430356249996994, 25.36562499938548498, 8.999999999999992895 ) ) ;
#2376=LINE ( 'NONE', #12040, #17207 ) ;
#2399=ADVANCED_FACE ( 'NONE', ( #5760 ), #19765, .T. ) ;
#2401=CARTESIAN_POINT ( 'NONE',  ( 3.735045420075836212E-15, 27.05312499938548498, 4.662447845253954171 ) ) ;
#2403=FACE_OUTER_BOUND ( 'NONE', #20273, .T. ) ;
#2415=CARTESIAN_POINT ( 'NONE',  ( 2.000000000000000888, 29.81874999877096855, 12.46410161513774817 ) ) ;
#2423=CARTESIAN_POINT ( 'NONE',  ( -1.071796769724487230, 27.77634618820330559, 4.999999999999992006 ) ) ;
#2447=CARTESIAN_POINT ( 'NONE',  ( 3.756430356250004099, 26.07812499938548356, 6.831223922626973533 ) ) ;
#2452=ORIENTED_EDGE ( 'NONE', *, *, #20965, .F. ) ;
#2463=CARTESIAN_POINT ( 'NONE',  ( -3.999999999999995559, 26.93124999877096926, 6.690598923241487306 ) ) ;
#2468=PRESENTATION_STYLE_ASSIGNMENT (( #2350 ) ) ;
#2473=AXIS2_PLACEMENT_3D ( 'NONE', #12395, #8347, #16079 ) ;
#2475=CARTESIAN_POINT ( 'NONE',  ( 3.735045420075836212E-15, 25.25312499938548427, 4.662447845253954171 ) ) ;
#2484=CARTESIAN_POINT ( 'NONE',  ( -1.999999999999998224, 28.00000000000000000, 12.46410161513774639 ) ) ;
#2493=ORIENTED_EDGE ( 'NONE', *, *, #3693, .F. ) ;
#2528=EDGE_LOOP ( 'NONE', ( #6641, #17739, #11163 ) ) ;
#2534=CARTESIAN_POINT ( 'NONE',  ( 1.878215178125000939, 27.31562499938548427, 12.25316411605952283 ) ) ;
#2536=AXIS2_PLACEMENT_3D ( 'NONE', #15735, #21999, #13642 ) ;
#2554=CARTESIAN_POINT ( 'NONE',  ( -3.756430356249997882, 25.96562499938548640, 11.16877607737301226 ) ) ;
#2569=DIRECTION ( 'NONE',  ( -0.000000000000000000, -1.000000000000000000, -0.000000000000000000 ) ) ;
#2586=CARTESIAN_POINT ( 'NONE',  ( -1.878215178124998497, 29.60312499938548569, 12.25316411605951927 ) ) ;
#2599=EDGE_CURVE ( 'NONE', #5942, #4195, #2627, .T. ) ;
#2615=VECTOR ( 'NONE', #13942, 1000.000000000000000 ) ;
#2618=CARTESIAN_POINT ( 'NONE',  ( 3.756430356250003655, 25.14062499938548356, 8.999999999999992895 ) ) ;
#2627=LINE ( 'NONE', #18454, #20438 ) ;
#2640=ORIENTED_EDGE ( 'NONE', *, *, #8385, .T. ) ;
#2671=CARTESIAN_POINT ( 'NONE',  ( 2.000000000000000888, 25.37500000000000000, 12.46410161513774817 ) ) ;
#2684=EDGE_LOOP ( 'NONE', ( #23658, #14103, #22454, #9448 ) ) ;
#2685=CARTESIAN_POINT ( 'NONE',  ( 2.672651547586948120E-15, 26.04062499938548925, 13.33755215474602984 ) ) ;
#2692=EDGE_CURVE ( 'NONE', #22640, #11825, #5350, .T. ) ;
#2701=DIRECTION ( 'NONE',  ( 0.000000000000000000, 0.000000000000000000, -1.000000000000000000 ) ) ;
#2710=CARTESIAN_POINT ( 'NONE',  ( -3.756430356249996994, 29.07812499938548356, 8.999999999999992895 ) ) ;
#2716=CARTESIAN_POINT ( 'NONE',  ( 3.834746474454188013E-15, 25.95624999877096428, 4.999999999999992006 ) ) ;
#2739=CARTESIAN_POINT ( 'NONE',  ( 3.756430356250003655, 28.29062499938548569, 8.999999999999992895 ) ) ;
#2755=ORIENTED_EDGE ( 'NONE', *, *, #2599, .F. ) ;
#2772=EDGE_CURVE ( 'NONE', #2907, #4929, #9413, .T. ) ;
#2789=CARTESIAN_POINT ( 'NONE',  ( -3.756430356249995661, 28.92812499938548143, 6.831223922626973533 ) ) ;
#2790=CARTESIAN_POINT ( 'NONE',  ( -3.999999999999995559, 28.28124999877096712, 6.690598923241487306 ) ) ;
#2806=CARTESIAN_POINT ( 'NONE',  ( 2.672651547586948120E-15, 25.59062499938548640, 13.33755215474602984 ) ) ;
#2833=CARTESIAN_POINT ( 'NONE',  ( 3.756430356250003655, 26.94062499938548427, 8.999999999999992895 ) ) ;
#2845=ADVANCED_FACE ( 'NONE', ( #17653 ), #23918, .T. ) ;
#2862=CARTESIAN_POINT ( 'NONE',  ( -1.878215178124995832, 28.44062499938548427, 5.746835883940462963 ) ) ;
#2867=CARTESIAN_POINT ( 'NONE',  ( -1.878215178124995832, 25.85312499938548569, 5.746835883940462963 ) ) ;
#2896=ADVANCED_FACE ( 'NONE', ( #3775 ), #25623, .T. ) ;
#2907=VERTEX_POINT ( 'NONE', #21951 ) ;
#2924=CARTESIAN_POINT ( 'NONE',  ( -1.999999999999998224, 25.75000000000000355, 12.46410161513774639 ) ) ;
#2925=CARTESIAN_POINT ( 'NONE',  ( 1.071796769724491227, 27.28615380933863577, 4.999999999999989342 ) ) ;
#2931=CARTESIAN_POINT ( 'NONE',  ( -1.071796769724488563, 28.46740381056766722, 12.99999999999999289 ) ) ;
#2942=CARTESIAN_POINT ( 'NONE',  ( -1.999999999999998224, 29.29374999877096997, 12.46410161513774639 ) ) ;
#2972=CARTESIAN_POINT ( 'NONE',  ( 3.756430356250002323, 28.70312499938548356, 11.16877607737301226 ) ) ;
#2987=EDGE_LOOP ( 'NONE', ( #21157, #16477, #16651, #17394 ) ) ;
#3001=CARTESIAN_POINT ( 'NONE',  ( -3.756430356249996105, 28.47812499938548569, 6.831223922626973533 ) ) ;
#3008=CARTESIAN_POINT ( 'NONE',  ( 3.735045420075836212E-15, 26.26562499938548356, 4.662447845253954171 ) ) ;
#3010=CARTESIAN_POINT ( 'NONE',  ( -1.071796769724493448, 29.57634618820329564, 4.999999999999995559 ) ) ;
#3012=LINE ( 'NONE', #19083, #140 ) ;
#3053=( BOUNDED_SURFACE ( )  B_SPLINE_SURFACE ( 1, 2, ( 
 ( #23602, #19669, #5561, #21389, #3589, #13275, #1630, #3469, #11441, #15754, #11307, #23717, #3329, #19413, #1506, #9477, #17455, #25425, #7512, #15506, #23473, #17590, #23987, #4487, #2017, #17978, #11946, #14181, #9985, #19916, #68, #24383, #18503, #18235, #3981, #22407, #16023, #16273, #2155, #12076, #20307, #6460, #24242, #12463, #10358, #12215, #10123, #16539, #20436, #14447, #8041, #2401, #16415, #5944, #12343, #195, #10238, #457, #2534, #10503, #18359, #8428, #4098, #6330, #591, #6070, #8557, #13930, #6191, #22151, #21898, #14053, #18122, #22019, #8168, #20050, #16147, #24108, #4236, #20184, #2283, #318, #8289, #14323, #22287, #4366, #25016, #3057, #10884, #8953, #708, #16927, #1214, #9195, #7105, #14705, #8676, #13129, #19006, #24895, #22806, #2789, #24501, #16657, #971, #14562, #832, #11026, #5153, #6850, #6973, #24624, #10753, #5015, #18884, #6580, #19122, #22543, #4623, #22928, #14953 ),
 ( #1089, #18743, #4883, #18623, #9063, #12606, #17045, #15090, #12856, #10631, #2671, #12997, #20833, #20581, #6710, #23068, #20977, #8809, #16802, #21099, #2924, #22683, #4768, #3177, #11143, #12739, #20710, #24768, #14833, #21605, #11801, #17561, #25536, #7621, #21357, #19776, #15607, #1603, #11660, #23576, #11413, #5773, #11271, #9573, #17697, #19637, #13757, #13518, #1872, #21487, #7361, #19256, #21736, #3562, #3820, #11536, #9715, #19503, #5654, #25157, #5270, #13636, #17431, #17183, #7240, #15219, #23692, #23185, #13248, #3682, #1743, #25666, #7745, #25397, #5391, #13382, #21217, #15728, #3298, #1356, #9333, #17317, #19387, #25280, #15339, #23307, #3441, #1480, #9451, #7484, #15473, #23442, #5532, #23961, #7866, #11919, #20155, #21871, #22375, #9834, #4203, #9955, #10331, #17817, #5911, #2255, #19889, #14149, #24348, #18088, #16117, #13899, #8008, #10087, #25782, #18209, #22115, #291, #8260, #6043, #12181 ) ),
 .UNSPECIFIED., .F., .F., .F. ) 
 B_SPLINE_SURFACE_WITH_KNOTS ( ( 2, 2 ),
 ( 3, 2, 2, 2, 2, 2, 2, 2, 2, 2, 2, 2, 2, 2, 2, 2, 2, 2, 2, 2, 2, 2, 2, 2, 2, 2, 2, 2, 2, 2, 2, 2, 2, 2, 2, 2, 2, 2, 2, 2, 2, 2, 2, 2, 2, 2, 2, 2, 2, 2, 2, 2, 2, 2, 2, 2, 2, 2, 2, 2, 3 ),
 ( 0.000000000000000000, 1.000000000000000000 ),
 ( 0.000000000000000000, 0.01666666666666666644, 0.03333333333333333287, 0.05000000000000000278, 0.06666666666666666574, 0.08333333333333332871, 0.1000000000000000056, 0.1166666666666666685, 0.1333333333333333315, 0.1499999999999999944, 0.1666666666666666574, 0.1833333333333333204, 0.2000000000000000111, 0.2166666666666666741, 0.2333333333333333370, 0.2500000000000000000, 0.2666666666666666630, 0.2833333333333333259, 0.2999999999999999889, 0.3166666666666666519, 0.3333333333333333148, 0.3499999999999999778, 0.3666666666666666408, 0.3833333333333333592, 0.4000000000000000222, 0.4166666666666666852, 0.4333333333333333481, 0.4500000000000000111, 0.4666666666666666741, 0.4833333333333333370, 0.5000000000000000000, 0.5166666666666667185, 0.5333333333333333259, 0.5500000000000000444, 0.5666666666666666519, 0.5833333333333333703, 0.5999999999999999778, 0.6166666666666666963, 0.6333333333333333037, 0.6500000000000000222, 0.6666666666666666297, 0.6833333333333333481, 0.6999999999999999556, 0.7166666666666666741, 0.7333333333333332815, 0.7500000000000000000, 0.7666666666666667185, 0.7833333333333333259, 0.8000000000000000444, 0.8166666666666666519, 0.8333333333333333703, 0.8499999999999999778, 0.8666666666666666963, 0.8833333333333333037, 0.9000000000000000222, 0.9166666666666666297, 0.9333333333333333481, 0.9499999999999999556, 0.9666666666666666741, 0.9833333333333332815, 1.000000000000000000 ),
 .UNSPECIFIED. ) 
 GEOMETRIC_REPRESENTATION_ITEM ( )  RATIONAL_B_SPLINE_SURFACE ( (
 ( 1.000000000000000000, 0.8660254037844387076, 1.000000000000000000, 0.8660254037844387076, 1.000000000000000000, 0.8660254037844387076, 1.000000000000000000, 0.8660254037844387076, 1.000000000000000000, 0.8660254037844387076, 1.000000000000000000, 0.8660254037844387076, 1.000000000000000000, 0.8660254037844387076, 1.000000000000000000, 0.8660254037844387076, 1.000000000000000000, 0.8660254037844387076, 1.000000000000000000, 0.8660254037844387076, 1.000000000000000000, 0.8660254037844387076, 1.000000000000000000, 0.8660254037844387076, 1.000000000000000000, 0.8660254037844387076, 1.000000000000000000, 0.8660254037844387076, 1.000000000000000000, 0.8660254037844387076, 1.000000000000000000, 0.8660254037844387076, 1.000000000000000000, 0.8660254037844387076, 1.000000000000000000, 0.8660254037844387076, 1.000000000000000000, 0.8660254037844387076, 1.000000000000000000, 0.8660254037844387076, 1.000000000000000000, 0.8660254037844387076, 1.000000000000000000, 0.8660254037844387076, 1.000000000000000000, 0.8660254037844387076, 1.000000000000000000, 0.8660254037844387076, 1.000000000000000000, 0.8660254037844387076, 1.000000000000000000, 0.8660254037844387076, 1.000000000000000000, 0.8660254037844387076, 1.000000000000000000, 0.8660254037844387076, 1.000000000000000000, 0.8660254037844387076, 1.000000000000000000, 0.8660254037844387076, 1.000000000000000000, 0.8660254037844387076, 1.000000000000000000, 0.8660254037844387076, 1.000000000000000000, 0.8660254037844387076, 1.000000000000000000, 0.8660254037844387076, 1.000000000000000000, 0.8660254037844387076, 1.000000000000000000, 0.8660254037844387076, 1.000000000000000000, 0.8660254037844387076, 1.000000000000000000, 0.8660254037844387076, 1.000000000000000000, 0.8660254037844387076, 1.000000000000000000, 0.8660254037844387076, 1.000000000000000000, 0.8660254037844387076, 1.000000000000000000, 0.8660254037844387076, 1.000000000000000000, 0.8660254037844387076, 1.000000000000000000, 0.8660254037844387076, 1.000000000000000000, 0.8660254037844387076, 1.000000000000000000, 0.8660254037844387076, 1.000000000000000000, 0.8660254037844387076, 1.000000000000000000, 0.8660254037844387076, 1.000000000000000000, 0.8660254037844387076, 1.000000000000000000, 0.8660254037844387076, 1.000000000000000000, 0.8660254037844387076, 1.000000000000000000, 0.8660254037844387076, 1.000000000000000000, 0.8660254037844387076, 1.000000000000000000, 0.8660254037844387076, 1.000000000000000000, 0.8660254037844387076, 1.000000000000000000, 0.8660254037844387076, 1.000000000000000000, 0.8660254037844387076, 1.000000000000000000, 0.8660254037844387076, 1.000000000000000000, 0.8660254037844387076, 1.000000000000000000, 0.8660254037844387076, 1.000000000000000000),
 ( 1.000000000000000000, 0.8660254037844387076, 1.000000000000000000, 0.8660254037844387076, 1.000000000000000000, 0.8660254037844387076, 1.000000000000000000, 0.8660254037844387076, 1.000000000000000000, 0.8660254037844387076, 1.000000000000000000, 0.8660254037844387076, 1.000000000000000000, 0.8660254037844387076, 1.000000000000000000, 0.8660254037844387076, 1.000000000000000000, 0.8660254037844387076, 1.000000000000000000, 0.8660254037844387076, 1.000000000000000000, 0.8660254037844387076, 1.000000000000000000, 0.8660254037844387076, 1.000000000000000000, 0.8660254037844387076, 1.000000000000000000, 0.8660254037844387076, 1.000000000000000000, 0.8660254037844387076, 1.000000000000000000, 0.8660254037844387076, 1.000000000000000000, 0.8660254037844387076, 1.000000000000000000, 0.8660254037844387076, 1.000000000000000000, 0.8660254037844387076, 1.000000000000000000, 0.8660254037844387076, 1.000000000000000000, 0.8660254037844387076, 1.000000000000000000, 0.8660254037844387076, 1.000000000000000000, 0.8660254037844387076, 1.000000000000000000, 0.8660254037844387076, 1.000000000000000000, 0.8660254037844387076, 1.000000000000000000, 0.8660254037844387076, 1.000000000000000000, 0.8660254037844387076, 1.000000000000000000, 0.8660254037844387076, 1.000000000000000000, 0.8660254037844387076, 1.000000000000000000, 0.8660254037844387076, 1.000000000000000000, 0.8660254037844387076, 1.000000000000000000, 0.8660254037844387076, 1.000000000000000000, 0.8660254037844387076, 1.000000000000000000, 0.8660254037844387076, 1.000000000000000000, 0.8660254037844387076, 1.000000000000000000, 0.8660254037844387076, 1.000000000000000000, 0.8660254037844387076, 1.000000000000000000, 0.8660254037844387076, 1.000000000000000000, 0.8660254037844387076, 1.000000000000000000, 0.8660254037844387076, 1.000000000000000000, 0.8660254037844387076, 1.000000000000000000, 0.8660254037844387076, 1.000000000000000000, 0.8660254037844387076, 1.000000000000000000, 0.8660254037844387076, 1.000000000000000000, 0.8660254037844387076, 1.000000000000000000, 0.8660254037844387076, 1.000000000000000000, 0.8660254037844387076, 1.000000000000000000, 0.8660254037844387076, 1.000000000000000000, 0.8660254037844387076, 1.000000000000000000, 0.8660254037844387076, 1.000000000000000000, 0.8660254037844387076, 1.000000000000000000, 0.8660254037844387076, 1.000000000000000000, 0.8660254037844387076, 1.000000000000000000, 0.8660254037844387076, 1.000000000000000000, 0.8660254037844387076, 1.000000000000000000, 0.8660254037844387076, 1.000000000000000000, 0.8660254037844387076, 1.000000000000000000, 0.8660254037844387076, 1.000000000000000000, 0.8660254037844387076, 1.000000000000000000, 0.8660254037844387076, 1.000000000000000000) ) ) 
 REPRESENTATION_ITEM ( '' )  SURFACE ( )  );
#3057=CARTESIAN_POINT ( 'NONE',  ( 3.735045420075836212E-15, 28.40312499938548640, 4.662447845253954171 ) ) ;
#3059=CARTESIAN_POINT ( 'NONE',  ( 1.859271017917182139E-15, 26.68750000000000000, 12.99999999999999289 ) ) ;
#3073=CARTESIAN_POINT ( 'NONE',  ( -1.071796769724490117, 26.93259618943234202, 4.999999999999992895 ) ) ;
#3074=CARTESIAN_POINT ( 'NONE',  ( 3.756430356250004099, 28.44062499938548783, 6.831223922626973533 ) ) ;
#3101=CARTESIAN_POINT ( 'NONE',  ( -1.878215178124995832, 26.64062499938548711, 5.746835883940462963 ) ) ;
#3107=CARTESIAN_POINT ( 'NONE',  ( -1.071796769724493448, 28.73259618943232852, 4.999999999999995559 ) ) ;
#3112=LINE ( 'NONE', #7411, #5393 ) ;
#3128=CARTESIAN_POINT ( 'NONE',  ( 1.878215178125000939, 29.11562499938548498, 12.25316411605952283 ) ) ;
#3135=CARTESIAN_POINT ( 'NONE',  ( -1.878215178124998497, 25.55312499938548854, 12.25316411605951927 ) ) ;
#3158=LINE ( 'NONE', #23170, #8697 ) ;
#3177=CARTESIAN_POINT ( 'NONE',  ( 4.000000000000001776, 25.86250000000000071, 11.30940107675849760 ) ) ;
#3178=CARTESIAN_POINT ( 'NONE',  ( -1.999999999999998224, 28.39374999877096784, 12.46410161513774639 ) ) ;
#3192=CARTESIAN_POINT ( 'NONE',  ( -1.878215178124998497, 27.80312499938548498, 12.25316411605951927 ) ) ;
#3214=CARTESIAN_POINT ( 'NONE',  ( -1.878215178124998497, 27.24062499938548498, 12.25316411605951927 ) ) ;
#3224=CARTESIAN_POINT ( 'NONE',  ( -1.878215178124995832, 26.30312499938548498, 5.746835883940462963 ) ) ;
#3240=CARTESIAN_POINT ( 'NONE',  ( 3.756430356250002323, 28.25312499938548427, 11.16877607737301403 ) ) ;
#3263=CARTESIAN_POINT ( 'NONE',  ( 1.859271017917182139E-15, 29.33124999877096428, 12.99999999999999289 ) ) ;
#3267=EDGE_CURVE ( 'NONE', #24971, #8379, #10211, .T. ) ;
#3294=CARTESIAN_POINT ( 'NONE',  ( 1.071796769724492338, 26.70759618943233704, 12.99999999999999467 ) ) ;
#3298=CARTESIAN_POINT ( 'NONE',  ( -3.999999999999996447, 27.92500000000000071, 8.999999999999992895 ) ) ;
#3304=DIRECTION ( 'NONE',  ( -0.000000000000000000, -1.000000000000000000, -0.000000000000000000 ) ) ;
#3320=CARTESIAN_POINT ( 'NONE',  ( 1.878215178125000939, 28.32812499938548711, 12.25316411605952283 ) ) ;
#3329=CARTESIAN_POINT ( 'NONE',  ( 3.756430356250003655, 25.59062499938548285, 8.999999999999992895 ) ) ;
#3331=CIRCLE ( 'NONE', #21294, 5.500000000000000000 ) ;
#3337=PRODUCT_CONTEXT ( 'NONE', #16627, 'mechanical' ) ;
#3347=CARTESIAN_POINT ( 'NONE',  ( 2.672651547586948120E-15, 26.82812499938548356, 13.33755215474602984 ) ) ;
#3354=CARTESIAN_POINT ( 'NONE',  ( -3.999999999999996447, 25.61874999877096926, 8.999999999999992895 ) ) ;
#3359=CARTESIAN_POINT ( 'NONE',  ( -1.878215178124998497, 26.90312499938548285, 12.25316411605951927 ) ) ;
#3376=CARTESIAN_POINT ( 'NONE',  ( 3.878215178125003604, 25.32343749907822783, 8.999999999999992895 ) ) ;
#3378=CARTESIAN_POINT ( 'NONE',  ( 1.071796769724494336, 25.75134618820330346, 12.99999999999999467 ) ) ;
#3401=CARTESIAN_POINT ( 'NONE',  ( -3.999999999999996447, 29.21874999877096712, 8.999999999999992895 ) ) ;
#3436=CARTESIAN_POINT ( 'NONE',  ( 4.000000000000001776, 26.76250000000000284, 11.30940107675849760 ) ) ;
#3441=CARTESIAN_POINT ( 'NONE',  ( 2.000000000000003997, 28.22500000000000142, 5.535898384862238508 ) ) ;
#3446=CARTESIAN_POINT ( 'NONE',  ( 3.469446951953614189E-15, 25.00000000000000000, 4.999999999999992006 ) ) ;
#3457=ORIENTED_EDGE ( 'NONE', *, *, #19557, .T. ) ;
#3459=CARTESIAN_POINT ( 'NONE',  ( -1.878215178124998497, 27.35312499938548569, 12.25316411605951927 ) ) ;
#3469=CARTESIAN_POINT ( 'NONE',  ( -3.756430356249997882, 25.40312499938548285, 11.16877607737301226 ) ) ;
#3474=VECTOR ( 'NONE', #11414, 1000.000000000000000 ) ;
#3512=CARTESIAN_POINT ( 'NONE',  ( 1.859271017917182139E-15, 26.68750000000000000, 12.99999999999999289 ) ) ;
#3518=CARTESIAN_POINT ( 'NONE',  ( 1.878215178125004048, 26.67812499938548498, 5.746835883940462963 ) ) ;
#3519=CARTESIAN_POINT ( 'NONE',  ( 1.859271017917182139E-15, 29.78124999877096712, 12.99999999999999289 ) ) ;
#3548=CARTESIAN_POINT ( 'NONE',  ( -1.999999999999998224, 25.75000000000000355, 12.46410161513774639 ) ) ;
#3562=CARTESIAN_POINT ( 'NONE',  ( -3.999999999999996003, 26.98750000000000426, 6.690598923241487306 ) ) ;
#3570=( BOUNDED_CURVE ( )  B_SPLINE_CURVE ( 2, ( #9009, #9269, #16988, #23134, #13191, #15404, #24954, #21162, #5090 ),
 .UNSPECIFIED., .F., .F. ) 
 B_SPLINE_CURVE_WITH_KNOTS ( ( 3, 2, 2, 2, 3 ),
 ( 0.7750000000000000222, 0.7833333333333333259, 0.8000000000000000444, 0.8166666666666666519, 0.8250000000000000666 ),
 .UNSPECIFIED. ) 
 CURVE ( )  GEOMETRIC_REPRESENTATION_ITEM ( )  RATIONAL_B_SPLINE_CURVE ( ( 0.9330127018922194093, 0.9330127018922194093, 1.000000000000000000, 0.8660254037844387076, 1.000000000000000000, 0.8660254037844387076, 1.000000000000000000, 0.9330127018922189652, 0.9330127018922194093 ) ) 
 REPRESENTATION_ITEM ( '' )  );
#3571=CARTESIAN_POINT ( 'NONE',  ( 1.859271017917182139E-15, 27.08124999877096784, 12.99999999999999289 ) ) ;
#3582=CARTESIAN_POINT ( 'NONE',  ( 1.878215178125004048, 26.67812499938548498, 5.746835883940462963 ) ) ;
#3589=CARTESIAN_POINT ( 'NONE',  ( -1.878215178124995832, 25.29062499938548569, 5.746835883940462963 ) ) ;
#3591=CYLINDRICAL_SURFACE ( 'NONE', #8823, 4.000000000000000000 ) ;
#3594=EDGE_CURVE ( 'NONE', #10718, #16937, #25595, .T. ) ;
#3604=CARTESIAN_POINT ( 'NONE',  ( 3.756430356250002323, 29.60312499938548569, 11.16877607737301226 ) ) ;
#3614=CARTESIAN_POINT ( 'NONE',  ( 3.756430356250002323, 26.56562499938548783, 11.16877607737301403 ) ) ;
#3635=CARTESIAN_POINT ( 'NONE',  ( 1.859271017917182139E-15, 28.93749999999999645, 12.99999999999999289 ) ) ;
#3636=CARTESIAN_POINT ( 'NONE',  ( -1.878215178124998497, 28.70312499938548356, 12.25316411605951927 ) ) ;
#3682=CARTESIAN_POINT ( 'NONE',  ( 2.620986760973688460E-15, 27.58750000000000213, 13.61880215351699874 ) ) ;
#3693=EDGE_CURVE ( 'NONE', #2271, #408, #181, .T. ) ;
#3696=ORIENTED_EDGE ( 'NONE', *, *, #14089, .F. ) ;
#3705=EDGE_CURVE ( 'NONE', #10879, #24971, #8191, .T. ) ;
#3720=EDGE_CURVE ( 'NONE', #21859, #24971, #11056, .T. ) ;
#3727=CARTESIAN_POINT ( 'NONE',  ( -3.756430356249996994, 29.41562499938548569, 8.999999999999992895 ) ) ;
#3732=VERTEX_POINT ( 'NONE', #2309 ) ;
#3733=CARTESIAN_POINT ( 'NONE',  ( 4.000000000000003553, 26.33124999877097139, 6.690598923241489970 ) ) ;
#3738=CARTESIAN_POINT ( 'NONE',  ( 2.672651547586948120E-15, 29.19062499938548427, 13.33755215474603162 ) ) ;
#3758=CYLINDRICAL_SURFACE ( 'NONE', #13434, 4.000000000000000000 ) ;
#3761=CARTESIAN_POINT ( 'NONE',  ( 2.000000000000000888, 25.76874999877096784, 12.46410161513774817 ) ) ;
#3767=CARTESIAN_POINT ( 'NONE',  ( -3.756430356249995661, 26.79062499938548925, 6.831223922626973533 ) ) ;
#3775=FACE_OUTER_BOUND ( 'NONE', #22218, .T. ) ;
#3787=CIRCLE ( 'NONE', #2536, 5.500000000000000000 ) ;
#3809=DIRECTION ( 'NONE',  ( 0.000000000000000000, 0.000000000000000000, -1.000000000000000000 ) ) ;
#3811=EDGE_CURVE ( 'NONE', #9446, #9323, #7124, .T. ) ;
#3819=ORIENTED_EDGE ( 'NONE', *, *, #11622, .F. ) ;
#3820=CARTESIAN_POINT ( 'NONE',  ( -3.999999999999996447, 27.02500000000000213, 8.999999999999992895 ) ) ;
#3836=ORIENTED_EDGE ( 'NONE', *, *, #841, .F. ) ;
#3840=VECTOR ( 'NONE', #9694, 999.9999999999998863 ) ;
#3843=CARTESIAN_POINT ( 'NONE',  ( -3.756430356249995661, 29.49062499938548498, 6.831223922626973533 ) ) ;
#3855=EDGE_CURVE ( 'NONE', #14526, #1168, #12890, .T. ) ;
#3874=CARTESIAN_POINT ( 'NONE',  ( -3.999999999999996003, 26.93124999877096926, 6.690598923241487306 ) ) ;
#3879=CARTESIAN_POINT ( 'NONE',  ( -3.756430356249996994, 29.52812499938548640, 8.999999999999992895 ) ) ;
#3886=( BOUNDED_CURVE ( )  B_SPLINE_CURVE ( 2, ( #18085, #14023, #19886, #1986, #1869 ),
 .UNSPECIFIED., .F., .F. ) 
 B_SPLINE_CURVE_WITH_KNOTS ( ( 3, 2, 3 ),
 ( 0.000000000000000000, 0.01666666666666666644, 0.02500000000000000486 ),
 .UNSPECIFIED. ) 
 CURVE ( )  GEOMETRIC_REPRESENTATION_ITEM ( )  RATIONAL_B_SPLINE_CURVE ( ( 1.000000000000000000, 0.8660254037844387076, 1.000000000000000000, 0.9330127018922194093, 0.9330127018922194093 ) ) 
 REPRESENTATION_ITEM ( '' )  );
#3904=CARTESIAN_POINT ( 'NONE',  ( 2.672651547586948120E-15, 27.84062499938548640, 13.33755215474602984 ) ) ;
#3925=EDGE_CURVE ( 'NONE', #22149, #21859, #6158, .T. ) ;
#3927=EDGE_CURVE ( 'NONE', #18460, #2271, #3886, .T. ) ;
#3959=DIRECTION ( 'NONE',  ( 0.000000000000000000, 0.000000000000000000, -1.000000000000000000 ) ) ;
#3968=ORIENTED_EDGE ( 'NONE', *, *, #17877, .F. ) ;
#3972=CARTESIAN_POINT ( 'NONE',  ( -1.071796769724487230, 25.97634618820330132, 4.999999999999992006 ) ) ;
#3981=CARTESIAN_POINT ( 'NONE',  ( 1.878215178125000939, 26.41562499938548214, 12.25316411605952283 ) ) ;
#3993=DIRECTION ( 'NONE',  ( -0.000000000000000000, -1.000000000000000000, -0.000000000000000000 ) ) ;
#3997=CARTESIAN_POINT ( 'NONE',  ( 4.000000000000001776, 27.60624999877096641, 11.30940107675849760 ) ) ;
#4000=ORIENTED_EDGE ( 'NONE', *, *, #3267, .F. ) ;
#4002=CARTESIAN_POINT ( 'NONE',  ( -3.756430356249996105, 28.14062499938548356, 6.831223922626973533 ) ) ;
#4023=CARTESIAN_POINT ( 'NONE',  ( -3.756430356249995661, 28.14062499938548356, 6.831223922626973533 ) ) ;
#4026=CARTESIAN_POINT ( 'NONE',  ( 4.000000000000003553, 25.19687499938548569, 8.999999999999992895 ) ) ;
#4045=DIRECTION ( 'NONE',  ( 0.000000000000000000, 0.000000000000000000, 1.000000000000000000 ) ) ;
#4047=CARTESIAN_POINT ( 'NONE',  ( -1.878215178124998497, 27.24062499938548498, 12.25316411605951927 ) ) ;
#4057=CARTESIAN_POINT ( 'NONE',  ( 4.000000000000003553, 28.63749999999999929, 6.690598923241489970 ) ) ;
#4079=CARTESIAN_POINT ( 'NONE',  ( 4.000000000000003553, 29.05000000000000071, 8.999999999999992895 ) ) ;
#4090=CARTESIAN_POINT ( 'NONE',  ( 3.756430356250003655, 29.75312499938548783, 8.999999999999992895 ) ) ;
#4098=CARTESIAN_POINT ( 'NONE',  ( 1.878215178125004048, 27.46562499938548640, 5.746835883940462963 ) ) ;
#4119=CARTESIAN_POINT ( 'NONE',  ( 2.000000000000000888, 28.01874999877096784, 12.46410161513774817 ) ) ;
#4123=EDGE_CURVE ( 'NONE', #22108, #1305, #4979, .T. ) ;
#4124=CARTESIAN_POINT ( 'NONE',  ( -1.878215178124995832, 28.55312499938548498, 5.746835883940462963 ) ) ;
#4126=DIRECTION ( 'NONE',  ( -0.000000000000000000, -1.000000000000000000, -0.000000000000000000 ) ) ;
#4138=CARTESIAN_POINT ( 'NONE',  ( -3.999999999999996447, 27.41874999877096641, 8.999999999999992895 ) ) ;
#4145=CARTESIAN_POINT ( 'NONE',  ( -3.137519842735244810E-15, 26.46249999999999858, 4.999999999999991118 ) ) ;
#4150=CARTESIAN_POINT ( 'NONE',  ( -3.756430356249997882, 29.56562499938549138, 11.16877607737301226 ) ) ;
#4179=CARTESIAN_POINT ( 'NONE',  ( 3.756430356250002323, 26.45312499938548356, 11.16877607737301403 ) ) ;
#4186=CARTESIAN_POINT ( 'NONE',  ( -1.071796769724487230, 27.83259618943233704, 4.999999999999992006 ) ) ;
#4189=DIRECTION ( 'NONE',  ( -0.000000000000000000, -1.000000000000000000, -0.000000000000000000 ) ) ;
#4195=VERTEX_POINT ( 'NONE', #24470 ) ;
#4198=ORIENTED_EDGE ( 'NONE', *, *, #2345, .T. ) ;
#4201=( GEOMETRIC_REPRESENTATION_CONTEXT ( 3 ) GLOBAL_UNCERTAINTY_ASSIGNED_CONTEXT ( ( #23009 ) ) GLOBAL_UNIT_ASSIGNED_CONTEXT ( ( #22125, #4213, #24359 ) ) REPRESENTATION_CONTEXT ( 'NONE', 'WORKASPACE' ) );
#4203=CARTESIAN_POINT ( 'NONE',  ( -1.999999999999995781, 28.75000000000000000, 5.535898384862237620 ) ) ;
#4213=( NAMED_UNIT ( * ) PLANE_ANGLE_UNIT ( ) SI_UNIT ( $, .RADIAN. ) );
#4223=EDGE_LOOP ( 'NONE', ( #21183, #19561, #14384, #830 ) ) ;
#4236=CARTESIAN_POINT ( 'NONE',  ( -3.756430356249996994, 28.06562499938548427, 8.999999999999992895 ) ) ;
#4259=CARTESIAN_POINT ( 'NONE',  ( -1.999999999999995781, 27.79374999877096997, 5.535898384862237620 ) ) ;
#4264=CARTESIAN_POINT ( 'NONE',  ( -3.756430356249997438, 29.11562499938548498, 11.16877607737301048 ) ) ;
#4291=CARTESIAN_POINT ( 'NONE',  ( -3.756430356249995661, 29.49062499938548498, 6.831223922626973533 ) ) ;
#4294=EDGE_LOOP ( 'NONE', ( #21564, #9350, #24727, #8153 ) ) ;
#4302=ORIENTED_EDGE ( 'NONE', *, *, #14089, .T. ) ;
#4315=CARTESIAN_POINT ( 'NONE',  ( -1.878215178124995832, 25.74062499938548498, 5.746835883940462963 ) ) ;
#4366=CARTESIAN_POINT ( 'NONE',  ( 3.756430356250004099, 28.32812499938548356, 6.831223922626973533 ) ) ;
#4380=CARTESIAN_POINT ( 'NONE',  ( 2.000000000000003997, 28.16874999877096997, 5.535898384862238508 ) ) ;
#4411=CARTESIAN_POINT ( 'NONE',  ( -3.756430356249997882, 25.85312499938548925, 11.16877607737301226 ) ) ;
#4429=CARTESIAN_POINT ( 'NONE',  ( -1.999999999999998224, 27.04374999877096641, 12.46410161513774639 ) ) ;
#4437=CARTESIAN_POINT ( 'NONE',  ( 3.756430356250003211, 26.97812499938547859, 6.831223922626973533 ) ) ;
#4472=CARTESIAN_POINT ( 'NONE',  ( 1.071796769724494558, 25.99240381056766580, 4.999999999999992895 ) ) ;
#4487=CARTESIAN_POINT ( 'NONE',  ( 3.756430356250002323, 26.00312499938548427, 11.16877607737301226 ) ) ;
#4491=CARTESIAN_POINT ( 'NONE',  ( -3.137519842735244810E-15, 26.91249999999999787, 4.999999999999991118 ) ) ;
#4504=CARTESIAN_POINT ( 'NONE',  ( -3.999999999999997335, 29.25624999877096499, 11.30940107675849404 ) ) ;
#4509=CARTESIAN_POINT ( 'NONE',  ( -3.999999999999995559, 28.73124999877096997, 6.690598923241487306 ) ) ;
#4511=CARTESIAN_POINT ( 'NONE',  ( -1.071796769724487230, 25.71115380933864003, 12.99999999999999467 ) ) ;
#4533=CARTESIAN_POINT ( 'NONE',  ( 3.756430356250004099, 26.52812499938548285, 6.831223922626973533 ) ) ;
#4540=CARTESIAN_POINT ( 'NONE',  ( -1.071796769724488563, 28.91740381056766651, 12.99999999999999289 ) ) ;
#4564=CARTESIAN_POINT ( 'NONE',  ( 1.878215178125004048, 26.11562499938548498, 5.746835883940462963 ) ) ;
#4621=ORIENTED_EDGE ( 'NONE', *, *, #8841, .T. ) ;
#4623=CARTESIAN_POINT ( 'NONE',  ( 1.878215178125000939, 29.56562499938548427, 12.25316411605952283 ) ) ;
#4646=CARTESIAN_POINT ( 'NONE',  ( -3.999999999999996447, 29.66874999877096997, 8.999999999999992895 ) ) ;
#4651=DIRECTION ( 'NONE',  ( -0.000000000000000000, -1.000000000000000000, -0.000000000000000000 ) ) ;
#4667=CIRCLE ( 'NONE', #9268, 4.000000000000000000 ) ;
#4676=CARTESIAN_POINT ( 'NONE',  ( 3.756430356250004099, 28.89062499938548356, 6.831223922626973533 ) ) ;
#4714=CARTESIAN_POINT ( 'NONE',  ( -3.756430356249997438, 29.45312499938548356, 11.16877607737301048 ) ) ;
#4756=LINE ( 'NONE', #5957, #2615 ) ;
#4758=ORIENTED_EDGE ( 'NONE', *, *, #25197, .T. ) ;
#4768=CARTESIAN_POINT ( 'NONE',  ( 2.000000000000000888, 25.82499999999999929, 12.46410161513774817 ) ) ;
#4775=CARTESIAN_POINT ( 'NONE',  ( 8.831537335106614961E-15, 26.23749999999999716, 12.99999999999999112 ) ) ;
#4782=CARTESIAN_POINT ( 'NONE',  ( 1.878215178125000939, 26.52812499938548285, 12.25316411605952283 ) ) ;
#4794=CARTESIAN_POINT ( 'NONE',  ( 1.859271017917182139E-15, 26.18124999877096570, 12.99999999999999289 ) ) ;
#4799=CYLINDRICAL_SURFACE ( 'NONE', #820, 4.000000000000000000 ) ;
#4808=CARTESIAN_POINT ( 'NONE',  ( -3.756430356249997882, 26.75312499938548427, 11.16877607737301226 ) ) ;
#4832=CARTESIAN_POINT ( 'NONE',  ( 1.878215178125000939, 29.56562499938548427, 12.25316411605952283 ) ) ;
#4838=CARTESIAN_POINT ( 'NONE',  ( 3.756430356250004099, 25.29062499938548569, 6.831223922626973533 ) ) ;
#4839=CARTESIAN_POINT ( 'NONE',  ( 8.831537335106614961E-15, 27.53124999877097068, 12.99999999999999112 ) ) ;
#4880=( BOUNDED_CURVE ( )  B_SPLINE_CURVE ( 2, ( #263, #17785, #22082, #8229, #6264, #24176, #20123, #16204, #25752 ),
 .UNSPECIFIED., .F., .F. ) 
 B_SPLINE_CURVE_WITH_KNOTS ( ( 3, 2, 2, 2, 3 ),
 ( 0.2250000000000000056, 0.2333333333333333370, 0.2500000000000000000, 0.2666666666666666630, 0.2750000000000000222 ),
 .UNSPECIFIED. ) 
 CURVE ( )  GEOMETRIC_REPRESENTATION_ITEM ( )  RATIONAL_B_SPLINE_CURVE ( ( 0.9330127018922194093, 0.9330127018922194093, 1.000000000000000000, 0.8660254037844387076, 1.000000000000000000, 0.8660254037844387076, 1.000000000000000000, 0.9330127018922191873, 0.9330127018922194093 ) ) 
 REPRESENTATION_ITEM ( '' )  );
#4883=CARTESIAN_POINT ( 'NONE',  ( 2.000000000000003997, 25.07499999999999929, 5.535898384862238508 ) ) ;
#4899=CARTESIAN_POINT ( 'NONE',  ( 1.878215178125000939, 25.62812499938548783, 12.25316411605952283 ) ) ;
#4904=CARTESIAN_POINT ( 'NONE',  ( 1.878215178125000939, 29.67812499938548498, 12.25316411605952283 ) ) ;
#4905=DIRECTION ( 'NONE',  ( -0.000000000000000000, -1.000000000000000000, -0.000000000000000000 ) ) ;
#4924=CARTESIAN_POINT ( 'NONE',  ( -3.756430356249996994, 28.06562499938548427, 8.999999999999992895 ) ) ;
#4929=VERTEX_POINT ( 'NONE', #6997 ) ;
#4954=UNCERTAINTY_MEASURE_WITH_UNIT (LENGTH_MEASURE( 1.000000000000000082E-05 ), #6137, 'distance_accuracy_value', 'NONE');
#4956=CARTESIAN_POINT ( 'NONE',  ( 3.735045420075836212E-15, 28.85312499938548569, 4.662447845253954171 ) ) ;
#4959=DIRECTION ( 'NONE',  ( -0.000000000000000000, -1.000000000000000000, -0.000000000000000000 ) ) ;
#4962=CARTESIAN_POINT ( 'NONE',  ( 3.756430356250002323, 25.66562499938548569, 11.16877607737301226 ) ) ;
#4974=ORIENTED_EDGE ( 'NONE', *, *, #16031, .F. ) ;
#4979=LINE ( 'NONE', #16623, #23902 ) ;
#5002=ORIENTED_EDGE ( 'NONE', *, *, #6339, .T. ) ;
#5015=CARTESIAN_POINT ( 'NONE',  ( -3.756430356249995661, 29.37812499938548427, 6.831223922626973533 ) ) ;
#5033=CARTESIAN_POINT ( 'NONE',  ( 3.735045420075836212E-15, 25.36562499938548498, 4.662447845253954171 ) ) ;
#5036=ORIENTED_EDGE ( 'NONE', *, *, #8279, .T. ) ;
#5065=CARTESIAN_POINT ( 'NONE',  ( -3.756430356249997882, 29.00312499938548072, 11.16877607737301226 ) ) ;
#5076=CARTESIAN_POINT ( 'NONE',  ( -1.878215178124995832, 27.20312499938548711, 5.746835883940462963 ) ) ;
#5077=AXIS2_PLACEMENT_3D ( 'NONE', #22809, #9198, #8955 ) ;
#5090=CARTESIAN_POINT ( 'NONE',  ( -1.057460391440397258E-14, 29.10624999877096641, 4.999999999999992006 ) ) ;
#5096=CARTESIAN_POINT ( 'NONE',  ( 2.672651547586948120E-15, 29.07812499938548356, 13.33755215474603162 ) ) ;
#5102=CARTESIAN_POINT ( 'NONE',  ( -1.878215178124995832, 26.30312499938548498, 5.746835883940462963 ) ) ;
#5104=PLANE ( 'NONE',  #11618 ) ;
#5153=CARTESIAN_POINT ( 'NONE',  ( 3.756430356250003655, 29.19062499938548072, 8.999999999999992895 ) ) ;
#5172=CARTESIAN_POINT ( 'NONE',  ( -3.756430356249997882, 27.76562499938549067, 11.16877607737301226 ) ) ;
#5182=LINE ( 'NONE', #12887, #11371 ) ;
#5194=CARTESIAN_POINT ( 'NONE',  ( -3.756430356249997882, 28.55312499938548498, 11.16877607737301226 ) ) ;
#5202=EDGE_CURVE ( 'NONE', #1305, #14690, #1865, .T. ) ;
#5205=CARTESIAN_POINT ( 'NONE',  ( -1.878215178124998497, 26.00312499938548783, 12.25316411605951927 ) ) ;
#5218=CARTESIAN_POINT ( 'NONE',  ( 3.735045420075836212E-15, 27.50312499938548427, 4.662447845253954171 ) ) ;
#5230=CARTESIAN_POINT ( 'NONE',  ( 3.756430356250003655, 29.69687499938548569, 8.999999999999992895 ) ) ;
#5256=CARTESIAN_POINT ( 'NONE',  ( -1.071796769724488563, 25.76740381056766793, 12.99999999999999289 ) ) ;
#5270=CARTESIAN_POINT ( 'NONE',  ( 4.000000000000003553, 27.25000000000000000, 8.999999999999992895 ) ) ;
#5273=CARTESIAN_POINT ( 'NONE',  ( 1.071796769724491227, 26.44240381056766509, 4.999999999999989342 ) ) ;
#5287=CARTESIAN_POINT ( 'NONE',  ( 3.756430356250004099, 27.99062499938548498, 6.831223922626973533 ) ) ;
#5312=CARTESIAN_POINT ( 'NONE',  ( -3.756430356249995661, 28.47812499938548569, 6.831223922626973533 ) ) ;
#5322=CARTESIAN_POINT ( 'NONE',  ( 3.735045420075836212E-15, 25.81562499938548783, 4.662447845253954171 ) ) ;
#5349=CARTESIAN_POINT ( 'NONE',  ( 4.000000000000003553, 27.25000000000000000, 8.999999999999992895 ) ) ;
#5350=LINE ( 'NONE', #24854, #10861 ) ;
#5359=CARTESIAN_POINT ( 'NONE',  ( -1.057460391440397258E-14, 29.10624999877096641, 4.999999999999992006 ) ) ;
#5371=CYLINDRICAL_SURFACE ( 'NONE', #21726, 4.000000000000000000 ) ;
#5391=CARTESIAN_POINT ( 'NONE',  ( 2.000000000000003997, 27.77500000000000213, 5.535898384862238508 ) ) ;
#5393=VECTOR ( 'NONE', #23364, 1000.000000000000000 ) ;
#5396=CARTESIAN_POINT ( 'NONE',  ( 8.831537335106614961E-15, 26.23749999999999716, 12.99999999999999112 ) ) ;
#5402=EDGE_CURVE ( 'NONE', #20971, #12396, #4880, .T. ) ;
#5418=CARTESIAN_POINT ( 'NONE',  ( -1.878215178124998497, 28.25312499938548427, 12.25316411605951927 ) ) ;
#5426=CARTESIAN_POINT ( 'NONE',  ( 1.626862140677534194E-14, 28.43124999877096570, 12.99999999999999289 ) ) ;
#5441=CARTESIAN_POINT ( 'NONE',  ( 2.672651547586948120E-15, 29.07812499938548001, 13.33755215474602984 ) ) ;
#5450=CARTESIAN_POINT ( 'NONE',  ( 2.000000000000000888, 29.42500000000000071, 12.46410161513774817 ) ) ;
#5452=CARTESIAN_POINT ( 'NONE',  ( 1.878215178125004048, 26.67812499938548498, 5.746835883940462963 ) ) ;
#5476=CARTESIAN_POINT ( 'NONE',  ( 3.756430356250004099, 28.44062499938548783, 6.831223922626973533 ) ) ;
#5529=CIRCLE ( 'NONE', #7191, 4.000000000000000000 ) ;
#5532=CARTESIAN_POINT ( 'NONE',  ( -1.999999999999998224, 28.44999999999999929, 12.46410161513774639 ) ) ;
#5552=CARTESIAN_POINT ( 'NONE',  ( 3.735045420075836212E-15, 28.96562499938548640, 4.662447845253954171 ) ) ;
#5561=CARTESIAN_POINT ( 'NONE',  ( 1.878215178125004048, 25.21562499938548285, 5.746835883940462963 ) ) ;
#5577=CARTESIAN_POINT ( 'NONE',  ( 1.071796769724494558, 28.24240381056766580, 4.999999999999992895 ) ) ;
#5582=CARTESIAN_POINT ( 'NONE',  ( 4.000000000000003553, 25.84374999877096712, 8.999999999999992895 ) ) ;
#5584=CARTESIAN_POINT ( 'NONE',  ( 1.859271017917182139E-15, 29.38749999999999929, 12.99999999999999289 ) ) ;
#5609=CARTESIAN_POINT ( 'NONE',  ( 3.735045420075836212E-15, 28.06562499938548427, 4.662447845253954171 ) ) ;
#5612=ORIENTED_EDGE ( 'NONE', *, *, #25472, .F. ) ;
#5638=CYLINDRICAL_SURFACE ( 'NONE', #23480, 4.000000000000000000 ) ;
#5654=CARTESIAN_POINT ( 'NONE',  ( 2.000000000000000888, 27.17500000000000071, 12.46410161513774817 ) ) ;
#5668=VERTEX_POINT ( 'NONE', #4794 ) ;
#5673=CARTESIAN_POINT ( 'NONE',  ( -1.878215178124995832, 28.10312499938548569, 5.746835883940462963 ) ) ;
#5674=CARTESIAN_POINT ( 'NONE',  ( 4.000000000000003553, 28.09374999877097068, 8.999999999999992895 ) ) ;
#5689=CARTESIAN_POINT ( 'NONE',  ( 2.000000000000000888, 28.97500000000000142, 12.46410161513774817 ) ) ;
#5694=CARTESIAN_POINT ( 'NONE',  ( 2.000000000000003997, 29.51874999877096784, 5.535898384862238508 ) ) ;
#5699=CARTESIAN_POINT ( 'NONE',  ( 2.000000000000003997, 25.91874999877096997, 5.535898384862238508 ) ) ;
#5703=CARTESIAN_POINT ( 'NONE',  ( 1.878215178125004048, 27.57812499938548711, 5.746835883940462963 ) ) ;
#5725=CARTESIAN_POINT ( 'NONE',  ( 3.735045420075836212E-15, 28.51562499938549067, 4.662447845253954171 ) ) ;
#5726=ADVANCED_FACE ( 'NONE', ( #16691 ), #6489, .T. ) ;
#5727=DIRECTION ( 'NONE',  ( 0.000000000000000000, 0.000000000000000000, -1.000000000000000000 ) ) ;
#5760=FACE_OUTER_BOUND ( 'NONE', #20731, .T. ) ;
#5773=CARTESIAN_POINT ( 'NONE',  ( -3.999999999999996003, 26.53750000000000142, 6.690598923241487306 ) ) ;
#5803=ORIENTED_EDGE ( 'NONE', *, *, #11589, .F. ) ;
#5821=CARTESIAN_POINT ( 'NONE',  ( 2.000000000000000888, 28.07500000000000284, 12.46410161513774817 ) ) ;
#5827=CARTESIAN_POINT ( 'NONE',  ( 3.752267015613588906E-15, 27.30624999877097281, 4.381197846482986158 ) ) ;
#5831=CARTESIAN_POINT ( 'NONE',  ( -1.878215178124995832, 29.45312499938548356, 5.746835883940462963 ) ) ;
#5859=CARTESIAN_POINT ( 'NONE',  ( -3.756430356249995661, 27.69062499938548427, 6.831223922626973533 ) ) ;
#5875=DIRECTION ( 'NONE',  ( -0.000000000000000000, -1.000000000000000000, -0.000000000000000000 ) ) ;
#5884=( NAMED_UNIT ( * ) SI_UNIT ( $, .STERADIAN. ) SOLID_ANGLE_UNIT ( ) );
#5890=DIRECTION ( 'NONE',  ( -0.000000000000000000, -1.000000000000000000, -0.000000000000000000 ) ) ;
#5898=ORIENTED_EDGE ( 'NONE', *, *, #24116, .F. ) ;
#5911=CARTESIAN_POINT ( 'NONE',  ( -1.999999999999998224, 28.90000000000000213, 12.46410161513774639 ) ) ;
#5936=CARTESIAN_POINT ( 'NONE',  ( 3.756430356250002323, 29.26562499938548356, 11.16877607737301226 ) ) ;
#5942=VERTEX_POINT ( 'NONE', #25189 ) ;
#5944=CARTESIAN_POINT ( 'NONE',  ( -3.756430356249995661, 27.12812499938548427, 6.831223922626973533 ) ) ;
#5954=CARTESIAN_POINT ( 'NONE',  ( -1.999999999999995781, 27.40000000000000213, 5.535898384862237620 ) ) ;
#5957=CARTESIAN_POINT ( 'NONE',  ( 3.959305671612554781E-15, 40.00000000000000000, 12.99999999999999289 ) ) ;
#5961=CARTESIAN_POINT ( 'NONE',  ( -3.999999999999996447, 25.22500000000000142, 8.999999999999992895 ) ) ;
#5964=ORIENTED_EDGE ( 'NONE', *, *, #3925, .T. ) ;
#5965=CARTESIAN_POINT ( 'NONE',  ( 4.000000000000001776, 27.15624999877097423, 11.30940107675849760 ) ) ;
#5969=CARTESIAN_POINT ( 'NONE',  ( -3.756430356249996105, 29.04062499938548569, 6.831223922626973533 ) ) ;
#5992=CARTESIAN_POINT ( 'NONE',  ( 3.756430356250002323, 27.91562499938548569, 11.16877607737301226 ) ) ;
#5995=MECHANICAL_DESIGN_GEOMETRIC_PRESENTATION_REPRESENTATION('',(#8922),#15605);
#5999=CARTESIAN_POINT ( 'NONE',  ( 3.834746474454188013E-15, 25.56250000000000000, 4.999999999999992006 ) ) ;
#6017=PLANE ( 'NONE',  #14666 ) ;
#6020=CARTESIAN_POINT ( 'NONE',  ( 3.756430356250003211, 26.52812499938548285, 6.831223922626973533 ) ) ;
#6036=VERTEX_POINT ( 'NONE', #8044 ) ;
#6043=CARTESIAN_POINT ( 'NONE',  ( 4.000000000000001776, 29.46250000000000568, 11.30940107675849760 ) ) ;
#6053=CARTESIAN_POINT ( 'NONE',  ( -3.999999999999995559, 29.23750000000000071, 6.690598923241487306 ) ) ;
#6063=CARTESIAN_POINT ( 'NONE',  ( -1.878215178124998497, 29.60312499938548569, 12.25316411605951927 ) ) ;
#6070=CARTESIAN_POINT ( 'NONE',  ( -3.756430356249995661, 27.57812499938548356, 6.831223922626973533 ) ) ;
#6080=( BOUNDED_CURVE ( )  B_SPLINE_CURVE ( 2, ( #17579, #57, #9976, #9469, #7885 ),
 .UNSPECIFIED., .F., .F. ) 
 B_SPLINE_CURVE_WITH_KNOTS ( ( 3, 2, 3 ),
 ( 0.9749999999999999778, 0.9833333333333332815, 1.000000000000000000 ),
 .UNSPECIFIED. ) 
 CURVE ( )  GEOMETRIC_REPRESENTATION_ITEM ( )  RATIONAL_B_SPLINE_CURVE ( ( 0.9330127018922194093, 0.9330127018922194093, 1.000000000000000000, 0.8660254037844387076, 1.000000000000000000 ) ) 
 REPRESENTATION_ITEM ( '' )  );
#6085=ORIENTED_EDGE ( 'NONE', *, *, #24897, .T. ) ;
#6086=CARTESIAN_POINT ( 'NONE',  ( -1.999999999999995781, 27.34374999877097068, 5.535898384862237620 ) ) ;
#6090=CARTESIAN_POINT ( 'NONE',  ( 3.735045420075836212E-15, 28.06562499938548427, 4.662447845253954171 ) ) ;
#6101=ADVANCED_FACE ( 'NONE', ( #17724 ), #3591, .T. ) ;
#6115=CARTESIAN_POINT ( 'NONE',  ( -1.878215178124995832, 29.45312499938548356, 5.746835883940462963 ) ) ;
#6137=( LENGTH_UNIT ( ) NAMED_UNIT ( * ) SI_UNIT ( .MILLI., .METRE. ) );
#6141=CARTESIAN_POINT ( 'NONE',  ( -1.878215178124995832, 25.29062499938548569, 5.746835883940462963 ) ) ;
#6158=LINE ( 'NONE', #17815, #6300 ) ;
#6173=CARTESIAN_POINT ( 'NONE',  ( 2.000000000000003997, 29.12500000000000000, 5.535898384862238508 ) ) ;
#6183=CARTESIAN_POINT ( 'NONE',  ( -1.878215178124998497, 29.15312499938548640, 12.25316411605951927 ) ) ;
#6191=CARTESIAN_POINT ( 'NONE',  ( -1.878215178124998497, 27.69062499938548427, 12.25316411605951927 ) ) ;
#6207=CARTESIAN_POINT ( 'NONE',  ( -1.071796769724487230, 25.13259618943233420, 4.999999999999992006 ) ) ;
#6211=CARTESIAN_POINT ( 'NONE',  ( -1.999999999999998224, 28.84374999877096712, 12.46410161513774639 ) ) ;
#6215=CARTESIAN_POINT ( 'NONE',  ( 3.756430356250003655, 27.95312499938548711, 8.999999999999992895 ) ) ;
#6217=CARTESIAN_POINT ( 'NONE',  ( 3.369928719974892281E-15, 25.50624999877096855, 4.999999999999992006 ) ) ;
#6231=( BOUNDED_CURVE ( )  B_SPLINE_CURVE ( 2, ( #8974, #1110, #17071, #25043, #24917, #7133, #24520, #16949, #21119 ),
 .UNSPECIFIED., .F., .F. ) 
 B_SPLINE_CURVE_WITH_KNOTS ( ( 3, 2, 2, 2, 3 ),
 ( 0.1749999999999999889, 0.1833333333333333204, 0.2000000000000000111, 0.2166666666666666741, 0.2250000000000000056 ),
 .UNSPECIFIED. ) 
 CURVE ( )  GEOMETRIC_REPRESENTATION_ITEM ( )  RATIONAL_B_SPLINE_CURVE ( ( 0.9330127018922194093, 0.9330127018922194093, 1.000000000000000000, 0.8660254037844387076, 1.000000000000000000, 0.8660254037844387076, 1.000000000000000000, 0.9330127018922194093, 0.9330127018922194093 ) ) 
 REPRESENTATION_ITEM ( '' )  );
#6235=AXIS2_PLACEMENT_3D ( 'NONE', #11909, #21724, #3809 ) ;
#6244=CARTESIAN_POINT ( 'NONE',  ( 1.878215178125000939, 25.51562499938548356, 12.25316411605952283 ) ) ;
#6255=ORIENTED_EDGE ( 'NONE', *, *, #21074, .T. ) ;
#6264=CARTESIAN_POINT ( 'NONE',  ( -3.999999999999996447, 26.51874999877097139, 8.999999999999992895 ) ) ;
#6271=ADVANCED_FACE ( 'NONE', ( #2403 ), #24627, .T. ) ;
#6274=CARTESIAN_POINT ( 'NONE',  ( 2.672651547586948120E-15, 27.27812499938548640, 13.33755215474603162 ) ) ;
#6295=ORIENTED_EDGE ( 'NONE', *, *, #16004, .F. ) ;
#6300=VECTOR ( 'NONE', #9953, 1000.000000000000000 ) ;
#6319=ORIENTED_EDGE ( 'NONE', *, *, #1907, .F. ) ;
#6320=CARTESIAN_POINT ( 'NONE',  ( 2.000000000000003997, 25.07499999999999929, 5.535898384862238508 ) ) ;
#6324=EDGE_CURVE ( 'NONE', #14520, #18733, #18892, .T. ) ;
#6330=CARTESIAN_POINT ( 'NONE',  ( 3.735045420075836212E-15, 27.50312499938548783, 4.662447845253954171 ) ) ;
#6339=EDGE_CURVE ( 'NONE', #18733, #14017, #18942, .T. ) ;
#6344=CARTESIAN_POINT ( 'NONE',  ( -1.071796769724487230, 25.31740381056767220, 12.99999999999999467 ) ) ;
#6345=EDGE_CURVE ( 'NONE', #16937, #23824, #1741, .T. ) ;
#6348=CARTESIAN_POINT ( 'NONE',  ( 4.000000000000003553, 26.74374999877096926, 8.999999999999992895 ) ) ;
#6353=CARTESIAN_POINT ( 'NONE',  ( -1.999999999999995781, 28.69374999877096855, 5.535898384862237620 ) ) ;
#6357=CARTESIAN_POINT ( 'NONE',  ( -1.999999999999995781, 27.79374999877096997, 5.535898384862237620 ) ) ;
#6373=CARTESIAN_POINT ( 'NONE',  ( 5.577813053751546416E-15, 25.33750000000000213, 12.99999999999999289 ) ) ;
#6379=CARTESIAN_POINT ( 'NONE',  ( 1.878215178125000939, 25.96562499938548285, 12.25316411605952283 ) ) ;
#6400=( BOUNDED_CURVE ( )  B_SPLINE_CURVE ( 2, ( #23183, #3294, #13378, #3436, #19383, #1477, #9449, #17558, #25533 ),
 .UNSPECIFIED., .F., .F. ) 
 B_SPLINE_CURVE_WITH_KNOTS ( ( 3, 2, 2, 2, 3 ),
 ( 0.3750000000000000000, 0.3833333333333333592, 0.4000000000000000222, 0.4166666666666666852, 0.4250000000000000444 ),
 .UNSPECIFIED. ) 
 CURVE ( )  GEOMETRIC_REPRESENTATION_ITEM ( )  RATIONAL_B_SPLINE_CURVE ( ( 0.9330127018922194093, 0.9330127018922194093, 1.000000000000000000, 0.8660254037844387076, 1.000000000000000000, 0.8660254037844387076, 1.000000000000000000, 0.9330127018922191873, 0.9330127018922194093 ) ) 
 REPRESENTATION_ITEM ( '' )  );
#6405=CARTESIAN_POINT ( 'NONE',  ( 2.672651547586948120E-15, 25.92812499938548498, 13.33755215474603162 ) ) ;
#6458=CARTESIAN_POINT ( 'NONE',  ( 2.000000000000003997, 28.61874999877096926, 5.535898384862238508 ) ) ;
#6460=CARTESIAN_POINT ( 'NONE',  ( -3.756430356249995661, 26.67812499938548498, 6.831223922626973533 ) ) ;
#6475=CARTESIAN_POINT ( 'NONE',  ( -1.878215178124995832, 25.40312499938548640, 5.746835883940462963 ) ) ;
#6482=CARTESIAN_POINT ( 'NONE',  ( -3.999999999999996447, 25.61874999877096926, 8.999999999999992895 ) ) ;
#6489=CYLINDRICAL_SURFACE ( 'NONE', #10154, 4.000000000000000000 ) ;
#6498=CARTESIAN_POINT ( 'NONE',  ( 4.000000000000001776, 27.66249999999999787, 11.30940107675849760 ) ) ;
#6500=CARTESIAN_POINT ( 'NONE',  ( 1.878215178125004048, 26.11562499938548498, 5.746835883940462963 ) ) ;
#6528=CARTESIAN_POINT ( 'NONE',  ( -3.756430356249996994, 26.26562499938548711, 8.999999999999992895 ) ) ;
#6553=DIRECTION ( 'NONE',  ( -0.000000000000000000, -1.000000000000000000, -0.000000000000000000 ) ) ;
#6580=CARTESIAN_POINT ( 'NONE',  ( -3.756430356249997882, 29.45312499938548356, 11.16877607737301226 ) ) ;
#6596=CARTESIAN_POINT ( 'NONE',  ( -1.999999999999995781, 29.59374999877096712, 5.535898384862237620 ) ) ;
#6621=CARTESIAN_POINT ( 'NONE',  ( 2.000000000000000888, 27.62500000000000000, 12.46410161513774817 ) ) ;
#6623=CARTESIAN_POINT ( 'NONE',  ( 3.735045420075836212E-15, 25.70312499938548001, 4.662447845253954171 ) ) ;
#6641=ORIENTED_EDGE ( 'NONE', *, *, #21998, .F. ) ;
#6656=CARTESIAN_POINT ( 'NONE',  ( 3.756430356250002323, 27.80312499938548143, 11.16877607737301403 ) ) ;
#6679=VECTOR ( 'NONE', #6553, 1000.000000000000000 ) ;
#6701=CARTESIAN_POINT ( 'NONE',  ( 4.000000000000003553, 25.00000000000000000, 8.999999999999992895 ) ) ;
#6706=VECTOR ( 'NONE', #4126, 1000.000000000000000 ) ;
#6710=CARTESIAN_POINT ( 'NONE',  ( 2.000000000000003997, 25.52500000000000213, 5.535898384862238508 ) ) ;
#6732=CARTESIAN_POINT ( 'NONE',  ( 3.756430356250004099, 25.29062499938548569, 6.831223922626973533 ) ) ;
#6764=CARTESIAN_POINT ( 'NONE',  ( 1.878215178125004048, 27.01562499938548711, 5.746835883940462963 ) ) ;
#6796=UNCERTAINTY_MEASURE_WITH_UNIT (LENGTH_MEASURE( 1.000000000000000082E-05 ), #9926, 'distance_accuracy_value', 'NONE');
#6824=CARTESIAN_POINT ( 'NONE',  ( 3.469446951953614189E-15, 40.00000000000000000, 4.999999999999992006 ) ) ;
#6850=CARTESIAN_POINT ( 'NONE',  ( 3.756430356250004099, 29.22812499938548925, 6.831223922626973533 ) ) ;
#6867=CARTESIAN_POINT ( 'NONE',  ( 2.000000000000003997, 29.51874999877096784, 5.535898384862238508 ) ) ;
#6872=CARTESIAN_POINT ( 'NONE',  ( 3.834746474454188013E-15, 28.65624999877096712, 4.999999999999992006 ) ) ;
#6883=FACE_OUTER_BOUND ( 'NONE', #18836, .T. ) ;
#6892=CARTESIAN_POINT ( 'NONE',  ( -3.756430356249996994, 28.51562499938548356, 8.999999999999992895 ) ) ;
#6895=CARTESIAN_POINT ( 'NONE',  ( 3.469446951953614189E-15, 25.00000000000000000, 8.999999999999992895 ) ) ;
#6897=CARTESIAN_POINT ( 'NONE',  ( -3.999999999999996447, 28.82499999999999929, 8.999999999999992895 ) ) ;
#6905=ORIENTED_EDGE ( 'NONE', *, *, #17877, .T. ) ;
#6918=VECTOR ( 'NONE', #1177, 1000.000000000000000 ) ;
#6919=CARTESIAN_POINT ( 'NONE',  ( -3.756430356249996994, 28.51562499938548356, 8.999999999999992895 ) ) ;
#6925=CARTESIAN_POINT ( 'NONE',  ( -3.756430356249997882, 25.96562499938548640, 11.16877607737301226 ) ) ;
#6926=CARTESIAN_POINT ( 'NONE',  ( 3.878215178125003604, 29.57031249969274356, 8.999999999999992895 ) ) ;
#6941=EDGE_LOOP ( 'NONE', ( #15565, #25746, #7742, #3457, #17141, #3836 ) ) ;
#6965=ORIENTED_EDGE ( 'NONE', *, *, #10618, .F. ) ;
#6973=CARTESIAN_POINT ( 'NONE',  ( 1.878215178125004048, 29.26562499938548356, 5.746835883940462963 ) ) ;
#6975=CARTESIAN_POINT ( 'NONE',  ( 2.000000000000003997, 27.26874999877097139, 5.535898384862238508 ) ) ;
#6986=CARTESIAN_POINT ( 'NONE',  ( 8.831537335106614961E-15, 27.13750000000000284, 12.99999999999999112 ) ) ;
#6987=CARTESIAN_POINT ( 'NONE',  ( -3.999999999999997335, 29.70624999877097139, 11.30940107675849404 ) ) ;
#6996=ORIENTED_EDGE ( 'NONE', *, *, #1068, .F. ) ;
#6997=CARTESIAN_POINT ( 'NONE',  ( 3.756430356250003655, 29.75312499938548783, 8.999999999999992895 ) ) ;
#7013=CARTESIAN_POINT ( 'NONE',  ( -3.756430356249995661, 28.92812499938548143, 6.831223922626973533 ) ) ;
#7016=DIRECTION ( 'NONE',  ( 0.000000000000000000, 1.000000000000000000, 0.000000000000000000 ) ) ;
#7024=CARTESIAN_POINT ( 'NONE',  ( 3.756430356250003655, 25.25312499938548427, 8.999999999999992895 ) ) ;
#7043=PRODUCT_DEFINITION_CONTEXT ( 'detailed design', #24801, 'design' ) ;
#7044=CARTESIAN_POINT ( 'NONE',  ( -1.878215178124998497, 29.49062499938548498, 12.25316411605951927 ) ) ;
#7051=CARTESIAN_POINT ( 'NONE',  ( -1.057460391440397258E-14, 29.55624999877096926, 4.999999999999992006 ) ) ;
#7084=( BOUNDED_CURVE ( )  B_SPLINE_CURVE ( 2, ( #12351, #8565, #14454, #8821, #10514, #22815, #20316, #20191, #4775 ),
 .UNSPECIFIED., .F., .F. ) 
 B_SPLINE_CURVE_WITH_KNOTS ( ( 3, 2, 2, 2, 3 ),
 ( 0.2250000000000000056, 0.2333333333333333370, 0.2500000000000000000, 0.2666666666666666630, 0.2750000000000000222 ),
 .UNSPECIFIED. ) 
 CURVE ( )  GEOMETRIC_REPRESENTATION_ITEM ( )  RATIONAL_B_SPLINE_CURVE ( ( 0.9330127018922194093, 0.9330127018922194093, 1.000000000000000000, 0.8660254037844387076, 1.000000000000000000, 0.8660254037844387076, 1.000000000000000000, 0.9330127018922191873, 0.9330127018922194093 ) ) 
 REPRESENTATION_ITEM ( '' )  );
#7085=CARTESIAN_POINT ( 'NONE',  ( 4.143002691484658293E-15, 46.00000000000000000, 14.49999999999999289 ) ) ;
#7105=CARTESIAN_POINT ( 'NONE',  ( 1.878215178125000939, 28.66562499938548569, 12.25316411605952283 ) ) ;
#7106=CARTESIAN_POINT ( 'NONE',  ( 4.000000000000001776, 27.15624999877097423, 11.30940107675849760 ) ) ;
#7107=VECTOR ( 'NONE', #13209, 1000.000000000000000 ) ;
#7113=CIRCLE ( 'NONE', #23815, 4.000000000000000000 ) ;
#7122=EDGE_CURVE ( 'NONE', #14017, #21478, #6400, .T. ) ;
#7124=CIRCLE ( 'NONE', #21738, 4.000000000000000000 ) ;
#7125=CARTESIAN_POINT ( 'NONE',  ( -1.878215178124995832, 26.75312499938548783, 5.746835883940462963 ) ) ;
#7133=CARTESIAN_POINT ( 'NONE',  ( 4.000000000000003553, 26.33124999877097139, 6.690598923241489970 ) ) ;
#7153=CARTESIAN_POINT ( 'NONE',  ( -3.756430356249995661, 28.02812499938548640, 6.831223922626973533 ) ) ;
#7163=CARTESIAN_POINT ( 'NONE',  ( 1.878215178125000939, 26.52812499938548285, 12.25316411605952283 ) ) ;
#7170=VERTEX_POINT ( 'NONE', #16906 ) ;
#7182=CARTESIAN_POINT ( 'NONE',  ( 3.756430356250002323, 28.70312499938548356, 11.16877607737301403 ) ) ;
#7186=FACE_OUTER_BOUND ( 'NONE', #6941, .T. ) ;
#7189=CARTESIAN_POINT ( 'NONE',  ( 3.756430356250003655, 25.70312499938548356, 8.999999999999992895 ) ) ;
#7191=AXIS2_PLACEMENT_3D ( 'NONE', #12812, #16999, #24963 ) ;
#7240=CARTESIAN_POINT ( 'NONE',  ( -1.999999999999995781, 27.40000000000000213, 5.535898384862237620 ) ) ;
#7245=( BOUNDED_CURVE ( )  B_SPLINE_CURVE ( 2, ( #25413, #3972, #25682, #13781, #21759, #11820, #19792, #16013, #11937 ),
 .UNSPECIFIED., .F., .F. ) 
 B_SPLINE_CURVE_WITH_KNOTS ( ( 3, 2, 2, 2, 3 ),
 ( 0.1250000000000000000, 0.1333333333333333315, 0.1499999999999999944, 0.1666666666666666574, 0.1749999999999999889 ),
 .UNSPECIFIED. ) 
 CURVE ( )  GEOMETRIC_REPRESENTATION_ITEM ( )  RATIONAL_B_SPLINE_CURVE ( ( 0.9330127018922194093, 0.9330127018922194093, 1.000000000000000000, 0.8660254037844387076, 1.000000000000000000, 0.8660254037844387076, 1.000000000000000000, 0.9330127018922194093, 0.9330127018922194093 ) ) 
 REPRESENTATION_ITEM ( '' )  );
#7259=CARTESIAN_POINT ( 'NONE',  ( 2.672651547586948120E-15, 27.39062499938548356, 13.33755215474602984 ) ) ;
#7284=CARTESIAN_POINT ( 'NONE',  ( 3.735045420075836212E-15, 27.50312499938548783, 4.662447845253954171 ) ) ;
#7289=ORIENTED_EDGE ( 'NONE', *, *, #5402, .T. ) ;
#7290=CARTESIAN_POINT ( 'NONE',  ( 4.000000000000003553, 25.39374999877096784, 8.999999999999992895 ) ) ;
#7295=CARTESIAN_POINT ( 'NONE',  ( -3.756430356249996105, 25.44062499938548427, 6.831223922626973533 ) ) ;
#7317=DIRECTION ( 'NONE',  ( -0.000000000000000000, -1.000000000000000000, -0.000000000000000000 ) ) ;
#7318=ORIENTED_EDGE ( 'NONE', *, *, #10618, .T. ) ;
#7361=CARTESIAN_POINT ( 'NONE',  ( 2.000000000000003997, 26.87500000000000355, 5.535898384862238508 ) ) ;
#7364=CARTESIAN_POINT ( 'NONE',  ( -1.999999999999995781, 26.50000000000000355, 5.535898384862237620 ) ) ;
#7372=ORIENTED_EDGE ( 'NONE', *, *, #16182, .F. ) ;
#7377=CARTESIAN_POINT ( 'NONE',  ( 3.735045420075836212E-15, 26.71562499938548640, 4.662447845253954171 ) ) ;
#7384=EDGE_CURVE ( 'NONE', #18733, #20971, #20412, .T. ) ;
#7401=CARTESIAN_POINT ( 'NONE',  ( -3.756430356249997882, 29.45312499938548356, 11.16877607737301226 ) ) ;
#7406=CARTESIAN_POINT ( 'NONE',  ( -1.999999999999998224, 26.14374999877096784, 12.46410161513774639 ) ) ;
#7411=CARTESIAN_POINT ( 'NONE',  ( 3.959305671612554781E-15, 40.00000000000000000, 12.99999999999999289 ) ) ;
#7438=FACE_OUTER_BOUND ( 'NONE', #21120, .T. ) ;
#7471=CARTESIAN_POINT ( 'NONE',  ( -3.999999999999997335, 25.71249999999999503, 11.30940107675849404 ) ) ;
#7484=CARTESIAN_POINT ( 'NONE',  ( -3.999999999999996003, 28.33750000000000213, 6.690598923241487306 ) ) ;
#7490=DIRECTION ( 'NONE',  ( -0.000000000000000000, -1.000000000000000000, -0.000000000000000000 ) ) ;
#7504=CARTESIAN_POINT ( 'NONE',  ( 1.878215178125004048, 28.92812499938548854, 5.746835883940462963 ) ) ;
#7505=CARTESIAN_POINT ( 'NONE',  ( 1.071796769724498999, 28.00134618820329635, 12.99999999999998757 ) ) ;
#7512=CARTESIAN_POINT ( 'NONE',  ( -3.756430356249996994, 25.81562499938548427, 8.999999999999992895 ) ) ;
#7519=CARTESIAN_POINT ( 'NONE',  ( 3.469446951953614189E-15, 40.00000000000000000, 8.999999999999992895 ) ) ;
#7527=CARTESIAN_POINT ( 'NONE',  ( 3.834746474454188013E-15, 28.26249999999999929, 4.999999999999992006 ) ) ;
#7538=CARTESIAN_POINT ( 'NONE',  ( 1.878215178125004048, 27.12812499938548783, 5.746835883940462963 ) ) ;
#7568=CARTESIAN_POINT ( 'NONE',  ( 3.756430356250002323, 27.46562499938548640, 11.16877607737301226 ) ) ;
#7621=CARTESIAN_POINT ( 'NONE',  ( 2.620986760973688460E-15, 26.23750000000000071, 13.61880215351699874 ) ) ;
#7633=CARTESIAN_POINT ( 'NONE',  ( 4.000000000000001776, 25.86250000000000071, 11.30940107675849760 ) ) ;
#7640=CARTESIAN_POINT ( 'NONE',  ( 3.735045420075836212E-15, 27.61562499938548498, 4.662447845253954171 ) ) ;
#7665=CARTESIAN_POINT ( 'NONE',  ( 1.071796769724492338, 29.35134618820330488, 12.99999999999999467 ) ) ;
#7670=CARTESIAN_POINT ( 'NONE',  ( 2.000000000000000888, 26.21874999877096712, 12.46410161513774817 ) ) ;
#7674=CARTESIAN_POINT ( 'NONE',  ( 1.878215178125004048, 28.02812499938548640, 5.746835883940462963 ) ) ;
#7685=CARTESIAN_POINT ( 'NONE',  ( -1.071796769724485454, 27.51115380933863719, 12.99999999999999467 ) ) ;
#7699=CARTESIAN_POINT ( 'NONE',  ( 3.756430356250004099, 27.99062499938548498, 6.831223922626973533 ) ) ;
#7704=CARTESIAN_POINT ( 'NONE',  ( 1.071796769724495668, 27.15759618943233633, 12.99999999999999112 ) ) ;
#7705=ADVANCED_FACE ( 'NONE', ( #19870 ), #5638, .T. ) ;
#7727=EDGE_CURVE ( 'NONE', #4195, #8387, #1720, .T. ) ;
#7742=ORIENTED_EDGE ( 'NONE', *, *, #9266, .T. ) ;
#7745=CARTESIAN_POINT ( 'NONE',  ( 4.000000000000003553, 27.70000000000000284, 8.999999999999992895 ) ) ;
#7749=DIRECTION ( 'NONE',  ( -0.000000000000000000, -1.000000000000000000, -0.000000000000000000 ) ) ;
#7777=DIRECTION ( 'NONE',  ( -0.000000000000000000, -1.000000000000000000, -0.000000000000000000 ) ) ;
#7792=CARTESIAN_POINT ( 'NONE',  ( 2.000000000000000888, 28.46874999877097068, 12.46410161513774817 ) ) ;
#7796=CARTESIAN_POINT ( 'NONE',  ( 3.735045420075836212E-15, 29.41562499938548569, 4.662447845253954171 ) ) ;
#7816=ORIENTED_EDGE ( 'NONE', *, *, #714, .F. ) ;
#7819=CARTESIAN_POINT ( 'NONE',  ( 1.878215178125000939, 27.42812499938548498, 12.25316411605952283 ) ) ;
#7824=CARTESIAN_POINT ( 'NONE',  ( 2.000000000000003997, 27.32500000000000284, 5.535898384862238508 ) ) ;
#7864=ORIENTED_EDGE ( 'NONE', *, *, #25119, .F. ) ;
#7866=CARTESIAN_POINT ( 'NONE',  ( 2.000000000000000888, 28.52500000000000213, 12.46410161513774817 ) ) ;
#7885=CARTESIAN_POINT ( 'NONE',  ( 4.000000000000003553, 29.89374999877096784, 8.999999999999992895 ) ) ;
#7888=CARTESIAN_POINT ( 'NONE',  ( 1.878215178125004048, 29.37812499938548783, 5.746835883940462963 ) ) ;
#7910=CARTESIAN_POINT ( 'NONE',  ( 3.834746474454188013E-15, 28.65624999877096712, 4.999999999999992006 ) ) ;
#7915=CARTESIAN_POINT ( 'NONE',  ( 4.000000000000003553, 29.48124999877097352, 6.690598923241489970 ) ) ;
#7916=CARTESIAN_POINT ( 'NONE',  ( -3.999999999999997335, 25.26249999999999929, 11.30940107675849404 ) ) ;
#7920=CARTESIAN_POINT ( 'NONE',  ( -1.999999999999998224, 27.49374999877096926, 12.46410161513774639 ) ) ;
#7924=CARTESIAN_POINT ( 'NONE',  ( -3.756430356249996994, 27.72812499938548569, 8.999999999999992895 ) ) ;
#7935=EDGE_CURVE ( 'NONE', #6036, #9323, #1044, .T. ) ;
#7952=CARTESIAN_POINT ( 'NONE',  ( -1.878215178124995832, 27.20312499938548711, 5.746835883940462963 ) ) ;
#7954=CARTESIAN_POINT ( 'NONE',  ( -1.999999999999998224, 29.74374999877096926, 12.46410161513774639 ) ) ;
#7976=CIRCLE ( 'NONE', #20490, 4.000000000000000000 ) ;
#7984=CARTESIAN_POINT ( 'NONE',  ( 1.878215178125000939, 26.86562499938548498, 12.25316411605952283 ) ) ;
#8008=CARTESIAN_POINT ( 'NONE',  ( -1.999999999999995781, 29.19999999999999929, 5.535898384862237620 ) ) ;
#8021=CARTESIAN_POINT ( 'NONE',  ( 1.071796769724492338, 25.80759618943233491, 12.99999999999999467 ) ) ;
#8029=ORIENTED_EDGE ( 'NONE', *, *, #1365, .F. ) ;
#8033=AXIS2_PLACEMENT_3D ( 'NONE', #21960, #5875, #25634 ) ;
#8035=EDGE_CURVE ( 'NONE', #16822, #7170, #5529, .T. ) ;
#8041=CARTESIAN_POINT ( 'NONE',  ( 1.878215178125004048, 27.01562499938548711, 5.746835883940462963 ) ) ;
#8044=CARTESIAN_POINT ( 'NONE',  ( 5.577813053751546416E-15, 25.33750000000000213, 12.99999999999999289 ) ) ;
#8058=CARTESIAN_POINT ( 'NONE',  ( -1.999999999999998224, 25.30000000000000426, 12.46410161513774639 ) ) ;
#8061=CARTESIAN_POINT ( 'NONE',  ( 4.000000000000001776, 28.50624999877096855, 11.30940107675849760 ) ) ;
#8066=CARTESIAN_POINT ( 'NONE',  ( 2.672651547586948120E-15, 27.39062499938548356, 13.33755215474603162 ) ) ;
#8084=CARTESIAN_POINT ( 'NONE',  ( 4.000000000000003553, 25.44999999999999929, 8.999999999999992895 ) ) ;
#8087=ORIENTED_EDGE ( 'NONE', *, *, #12336, .F. ) ;
#8091=CARTESIAN_POINT ( 'NONE',  ( -1.878215178124998497, 27.80312499938548498, 12.25316411605951927 ) ) ;
#8099=DIRECTION ( 'NONE',  ( 0.000000000000000000, 0.000000000000000000, -1.000000000000000000 ) ) ;
#8119=CARTESIAN_POINT ( 'NONE',  ( 1.878215178125004048, 27.01562499938548711, 5.746835883940462963 ) ) ;
#8128=CARTESIAN_POINT ( 'NONE',  ( 1.859271017917182139E-15, 28.48749999999999716, 12.99999999999999289 ) ) ;
#8151=CARTESIAN_POINT ( 'NONE',  ( 4.000000000000003553, 25.90000000000000213, 8.999999999999992895 ) ) ;
#8153=ORIENTED_EDGE ( 'NONE', *, *, #7384, .F. ) ;
#8168=CARTESIAN_POINT ( 'NONE',  ( 1.878215178125004048, 27.91562499938548569, 5.746835883940462963 ) ) ;
#8175=CARTESIAN_POINT ( 'NONE',  ( -1.071796769724487230, 27.38259618943233420, 4.999999999999992006 ) ) ;
#8184=CARTESIAN_POINT ( 'NONE',  ( -3.999999999999996003, 28.73124999877096641, 6.690598923241487306 ) ) ;
#8188=CARTESIAN_POINT ( 'NONE',  ( -3.756430356249997438, 28.66562499938548569, 11.16877607737301048 ) ) ;
#8191=LINE ( 'NONE', #14348, #9618 ) ;
#8207=CARTESIAN_POINT ( 'NONE',  ( 4.000000000000001776, 25.41250000000000142, 11.30940107675849760 ) ) ;
#8213=CARTESIAN_POINT ( 'NONE',  ( 3.756430356250004099, 25.17812499938548498, 6.831223922626973533 ) ) ;
#8215=EDGE_LOOP ( 'NONE', ( #9562, #12849 ) ) ;
#8218=ORIENTED_EDGE ( 'NONE', *, *, #6345, .T. ) ;
#8229=CARTESIAN_POINT ( 'NONE',  ( -3.999999999999995559, 26.48124999877096641, 6.690598923241487306 ) ) ;
#8239=CARTESIAN_POINT ( 'NONE',  ( 1.878215178125004048, 26.56562499938548427, 5.746835883940462963 ) ) ;
#8260=CARTESIAN_POINT ( 'NONE',  ( 2.000000000000000888, 29.42500000000000071, 12.46410161513774817 ) ) ;
#8279=EDGE_CURVE ( 'NONE', #14017, #12396, #4756, .T. ) ;
#8288=CARTESIAN_POINT ( 'NONE',  ( 1.626862140677534194E-14, 28.43124999877096570, 12.99999999999999289 ) ) ;
#8289=CARTESIAN_POINT ( 'NONE',  ( 1.878215178125000939, 28.21562499938548640, 12.25316411605952283 ) ) ;
#8308=CARTESIAN_POINT ( 'NONE',  ( -3.999999999999996447, 27.41874999877096641, 8.999999999999992895 ) ) ;
#8313=CARTESIAN_POINT ( 'NONE',  ( 3.959305671612554781E-15, 40.00000000000000000, 12.99999999999999289 ) ) ;
#8316=ORIENTED_EDGE ( 'NONE', *, *, #24116, .T. ) ;
#8337=CARTESIAN_POINT ( 'NONE',  ( -3.756430356249996994, 26.26562499938548711, 8.999999999999992895 ) ) ;
#8347=DIRECTION ( 'NONE',  ( -0.000000000000000000, -1.000000000000000000, -0.000000000000000000 ) ) ;
#8366=CARTESIAN_POINT ( 'NONE',  ( 3.735045420075836212E-15, 26.15312499938548285, 4.662447845253954171 ) ) ;
#8379=VERTEX_POINT ( 'NONE', #19492 ) ;
#8382=ORIENTED_EDGE ( 'NONE', *, *, #20992, .T. ) ;
#8385=EDGE_CURVE ( 'NONE', #11726, #23620, #23136, .T. ) ;
#8387=VERTEX_POINT ( 'NONE', #15325 ) ;
#8410=CARTESIAN_POINT ( 'NONE',  ( 2.000000000000003997, 25.97500000000000142, 5.535898384862238508 ) ) ;
#8419=ORIENTED_EDGE ( 'NONE', *, *, #3267, .T. ) ;
#8427=CARTESIAN_POINT ( 'NONE',  ( 4.000000000000003553, 28.54374999877096997, 8.999999999999992895 ) ) ;
#8428=CARTESIAN_POINT ( 'NONE',  ( 3.756430356250004099, 27.42812499938548143, 6.831223922626973533 ) ) ;
#8446=CARTESIAN_POINT ( 'NONE',  ( 4.000000000000001776, 29.40624999877096357, 11.30940107675849760 ) ) ;
#8451=ORIENTED_EDGE ( 'NONE', *, *, #6324, .T. ) ;
#8455=CARTESIAN_POINT ( 'NONE',  ( 5.577813053751546416E-15, 25.73124999877097352, 12.99999999999999289 ) ) ;
#8475=CARTESIAN_POINT ( 'NONE',  ( 1.878215178125004048, 25.21562499938548285, 5.746835883940462963 ) ) ;
#8485=FACE_OUTER_BOUND ( 'NONE', #23389, .T. ) ;
#8487=DIRECTION ( 'NONE',  ( -0.000000000000000000, -1.000000000000000000, -0.000000000000000000 ) ) ;
#8494=CARTESIAN_POINT ( 'NONE',  ( 1.859271017917182139E-15, 27.08124999877096784, 12.99999999999999289 ) ) ;
#8501=SURFACE_STYLE_FILL_AREA ( #20252 ) ;
#8507=CARTESIAN_POINT ( 'NONE',  ( 1.878215178125000939, 25.51562499938548356, 12.25316411605952283 ) ) ;
#8535=ADVANCED_FACE ( 'NONE', ( #19622 ), #9701, .T. ) ;
#8557=CARTESIAN_POINT ( 'NONE',  ( -3.756430356249996994, 27.61562499938548143, 8.999999999999992895 ) ) ;
#8565=CARTESIAN_POINT ( 'NONE',  ( -1.071796769724487230, 26.03259618943233278, 4.999999999999992006 ) ) ;
#8574=CARTESIAN_POINT ( 'NONE',  ( -3.756430356249996994, 25.47812499938548569, 8.999999999999992895 ) ) ;
#8579=CARTESIAN_POINT ( 'NONE',  ( 3.756430356250002323, 29.71562499938548640, 11.16877607737301403 ) ) ;
#8589=CARTESIAN_POINT ( 'NONE',  ( 3.469446951953614189E-15, 40.00000000000000000, 8.999999999999992895 ) ) ;
#8597=CARTESIAN_POINT ( 'NONE',  ( 3.735045420075836212E-15, 26.60312499938547859, 4.662447845253954171 ) ) ;
#8617=CARTESIAN_POINT ( 'NONE',  ( -1.999999999999995781, 26.89374999877097139, 5.535898384862237620 ) ) ;
#8626=CARTESIAN_POINT ( 'NONE',  ( 3.756430356250003655, 28.74062499938548498, 8.999999999999992895 ) ) ;
#8676=CARTESIAN_POINT ( 'NONE',  ( 3.756430356250003655, 28.74062499938548498, 8.999999999999992895 ) ) ;
#8690=CARTESIAN_POINT ( 'NONE',  ( 4.000000000000001776, 28.95624999877097494, 11.30940107675849760 ) ) ;
#8697=VECTOR ( 'NONE', #15452, 1000.000000000000000 ) ;
#8701=CARTESIAN_POINT ( 'NONE',  ( 1.859271017917182139E-15, 29.38749999999999929, 12.99999999999999289 ) ) ;
#8718=CARTESIAN_POINT ( 'NONE',  ( 2.672651547586948120E-15, 28.62812499938548783, 13.33755215474602984 ) ) ;
#8736=ORIENTED_EDGE ( 'NONE', *, *, #21132, .F. ) ;
#8750=CARTESIAN_POINT ( 'NONE',  ( 3.756430356250003655, 29.64062499938548356, 8.999999999999992895 ) ) ;
#8756=AXIS2_PLACEMENT_3D ( 'NONE', #25401, #3304, #19642 ) ;
#8784=EDGE_CURVE ( 'NONE', #21413, #23824, #22883, .T. ) ;
#8809=CARTESIAN_POINT ( 'NONE',  ( -3.999999999999996003, 25.63749999999999929, 6.690598923241487306 ) ) ;
#8821=CARTESIAN_POINT ( 'NONE',  ( -3.999999999999995559, 26.08749999999999503, 6.690598923241487306 ) ) ;
#8823=AXIS2_PLACEMENT_3D ( 'NONE', #25695, #7777, #18124 ) ;
#8832=CARTESIAN_POINT ( 'NONE',  ( 4.000000000000003553, 29.89374999877096784, 8.999999999999992895 ) ) ;
#8841=EDGE_CURVE ( 'NONE', #14526, #10206, #3012, .T. ) ;
#8862=CARTESIAN_POINT ( 'NONE',  ( 1.071796769724498999, 27.60759618943233207, 12.99999999999998757 ) ) ;
#8864=CARTESIAN_POINT ( 'NONE',  ( 1.878215178125000939, 27.76562499938548356, 12.25316411605952283 ) ) ;
#8871=CARTESIAN_POINT ( 'NONE',  ( -3.999999999999997335, 28.86250000000000071, 11.30940107675849404 ) ) ;
#8896=CARTESIAN_POINT ( 'NONE',  ( -3.756430356249996994, 28.96562499938548285, 8.999999999999992895 ) ) ;
#8922=STYLED_ITEM ( 'NONE', ( #2468 ), #22510 ) ;
#8934=( BOUNDED_CURVE ( )  B_SPLINE_CURVE ( 2, ( #18154, #13831, #17753, #12115, #4138, #22051, #19830, #7685, #14220 ),
 .UNSPECIFIED., .F., .F. ) 
 B_SPLINE_CURVE_WITH_KNOTS ( ( 3, 2, 2, 2, 3 ),
 ( 0.4250000000000000444, 0.4333333333333333481, 0.4500000000000000111, 0.4666666666666666741, 0.4750000000000000333 ),
 .UNSPECIFIED. ) 
 CURVE ( )  GEOMETRIC_REPRESENTATION_ITEM ( )  RATIONAL_B_SPLINE_CURVE ( ( 0.9330127018922194093, 0.9330127018922196314, 1.000000000000000000, 0.8660254037844387076, 1.000000000000000000, 0.8660254037844387076, 1.000000000000000000, 0.9330127018922191873, 0.9330127018922194093 ) ) 
 REPRESENTATION_ITEM ( '' )  );
#8945=( GEOMETRIC_REPRESENTATION_CONTEXT ( 3 ) GLOBAL_UNCERTAINTY_ASSIGNED_CONTEXT ( ( #4954 ) ) GLOBAL_UNIT_ASSIGNED_CONTEXT ( ( #6137, #12406, #2093 ) ) REPRESENTATION_CONTEXT ( 'NONE', 'WORKASPACE' ) );
#8948=ORIENTED_EDGE ( 'NONE', *, *, #12027, .T. ) ;
#8953=CARTESIAN_POINT ( 'NONE',  ( -3.756430356249995661, 28.47812499938548569, 6.831223922626973533 ) ) ;
#8955=DIRECTION ( 'NONE',  ( 0.000000000000000000, 0.000000000000000000, 1.000000000000000000 ) ) ;
#8958=CARTESIAN_POINT ( 'NONE',  ( 3.834746474454188013E-15, 28.26249999999999929, 4.999999999999992006 ) ) ;
#8967=CARTESIAN_POINT ( 'NONE',  ( 2.000000000000003997, 29.06874999877096855, 5.535898384862238508 ) ) ;
#8974=CARTESIAN_POINT ( 'NONE',  ( 1.859271017917182139E-15, 26.18124999877096570, 12.99999999999999289 ) ) ;
#8990=CARTESIAN_POINT ( 'NONE',  ( 1.878215178125000939, 26.86562499938548498, 12.25316411605952283 ) ) ;
#9009=CARTESIAN_POINT ( 'NONE',  ( 1.859271017917182139E-15, 28.88124999877096499, 12.99999999999999289 ) ) ;
#9029=ORIENTED_EDGE ( 'NONE', *, *, #1068, .T. ) ;
#9054=ORIENTED_EDGE ( 'NONE', *, *, #16182, .T. ) ;
#9063=CARTESIAN_POINT ( 'NONE',  ( -1.999999999999995781, 25.15000000000000213, 5.535898384862237620 ) ) ;
#9079=CARTESIAN_POINT ( 'NONE',  ( -3.756430356249995661, 27.69062499938548427, 6.831223922626973533 ) ) ;
#9096=CYLINDRICAL_SURFACE ( 'NONE', #19671, 4.000000000000000000 ) ;
#9102=CARTESIAN_POINT ( 'NONE',  ( 3.735045420075836212E-15, 27.05312499938548498, 4.662447845253954171 ) ) ;
#9108=CARTESIAN_POINT ( 'NONE',  ( 1.859271017917182139E-15, 28.93749999999999645, 12.99999999999999289 ) ) ;
#9113=CARTESIAN_POINT ( 'NONE',  ( 3.756430356250003655, 26.15312499938548640, 8.999999999999992895 ) ) ;
#9114=ORIENTED_EDGE ( 'NONE', *, *, #19557, .F. ) ;
#9126=CARTESIAN_POINT ( 'NONE',  ( 3.834746474454188013E-15, 27.81249999999999645, 4.999999999999992006 ) ) ;
#9132=CARTESIAN_POINT ( 'NONE',  ( 1.878215178125004048, 28.81562499938548427, 5.746835883940462963 ) ) ;
#9139=CARTESIAN_POINT ( 'NONE',  ( -1.878215178124998497, 26.45312499938548711, 12.25316411605951927 ) ) ;
#9185=ORIENTED_EDGE ( 'NONE', *, *, #16833, .T. ) ;
#9191=VECTOR ( 'NONE', #683, 1000.000000000000000 ) ;
#9195=CARTESIAN_POINT ( 'NONE',  ( 2.672651547586948120E-15, 28.62812499938548783, 13.33755215474602984 ) ) ;
#9198=DIRECTION ( 'NONE',  ( 0.000000000000000000, 1.000000000000000000, 0.000000000000000000 ) ) ;
#9202=CARTESIAN_POINT ( 'NONE',  ( -3.999999999999995559, 28.33750000000000213, 6.690598923241487306 ) ) ;
#9216=CARTESIAN_POINT ( 'NONE',  ( -3.756430356249995661, 26.79062499938548925, 6.831223922626973533 ) ) ;
#9246=CARTESIAN_POINT ( 'NONE',  ( 2.672651547586948120E-15, 28.17812499938548143, 13.33755215474602984 ) ) ;
#9252=CARTESIAN_POINT ( 'NONE',  ( 1.071796769724491227, 26.83615380933863293, 4.999999999999989342 ) ) ;
#9257=CARTESIAN_POINT ( 'NONE',  ( -3.756430356249996994, 26.37812499938548783, 8.999999999999992895 ) ) ;
#9266=EDGE_CURVE ( 'NONE', #9323, #8387, #7113, .T. ) ;
#9268=AXIS2_PLACEMENT_3D ( 'NONE', #18632, #14333, #14714 ) ;
#9269=CARTESIAN_POINT ( 'NONE',  ( 1.071796769724492338, 28.90134618820330203, 12.99999999999999467 ) ) ;
#9288=CARTESIAN_POINT ( 'NONE',  ( 4.000000000000003553, 27.28749999999999787, 6.690598923241489970 ) ) ;
#9289=DIRECTION ( 'NONE',  ( -0.000000000000000000, -1.000000000000000000, -0.000000000000000000 ) ) ;
#9317=CARTESIAN_POINT ( 'NONE',  ( 1.859271017917182139E-15, 25.78750000000000142, 12.99999999999999289 ) ) ;
#9323=VERTEX_POINT ( 'NONE', #11715 ) ;
#9333=CARTESIAN_POINT ( 'NONE',  ( -1.999999999999998224, 28.00000000000000000, 12.46410161513774639 ) ) ;
#9335=CARTESIAN_POINT ( 'NONE',  ( 1.071796769724495668, 26.25759618943233065, 12.99999999999999112 ) ) ;
#9350=ORIENTED_EDGE ( 'NONE', *, *, #20699, .T. ) ;
#9352=CARTESIAN_POINT ( 'NONE',  ( 3.735045420075836212E-15, 28.51562499938549067, 4.662447845253954171 ) ) ;
#9371=CARTESIAN_POINT ( 'NONE',  ( 8.831537335106614961E-15, 26.23749999999999716, 12.99999999999999112 ) ) ;
#9382=CARTESIAN_POINT ( 'NONE',  ( 1.071796769724495668, 26.65134618820330203, 12.99999999999999112 ) ) ;
#9406=CARTESIAN_POINT ( 'NONE',  ( -3.756430356249996994, 25.47812499938548569, 8.999999999999992895 ) ) ;
#9413=LINE ( 'NONE', #5230, #7107 ) ;
#9416=ORIENTED_EDGE ( 'NONE', *, *, #23543, .T. ) ;
#9446=VERTEX_POINT ( 'NONE', #3446 ) ;
#9448=ORIENTED_EDGE ( 'NONE', *, *, #20801, .F. ) ;
#9449=CARTESIAN_POINT ( 'NONE',  ( 2.000000000000003997, 26.87500000000000355, 5.535898384862238508 ) ) ;
#9451=CARTESIAN_POINT ( 'NONE',  ( -1.999999999999995781, 28.30000000000000071, 5.535898384862237620 ) ) ;
#9452=DIRECTION ( 'NONE',  ( 0.000000000000000000, 0.000000000000000000, -1.000000000000000000 ) ) ;
#9456=( BOUNDED_CURVE ( )  B_SPLINE_CURVE ( 2, ( #12946, #3010, #10979, #21175, #25867, #25351, #7954, #25737, #3519 ),
 .UNSPECIFIED., .F., .F. ) 
 B_SPLINE_CURVE_WITH_KNOTS ( ( 3, 2, 2, 2, 3 ),
 ( 0.9250000000000000444, 0.9333333333333333481, 0.9499999999999999556, 0.9666666666666666741, 0.9749999999999999778 ),
 .UNSPECIFIED. ) 
 CURVE ( )  GEOMETRIC_REPRESENTATION_ITEM ( )  RATIONAL_B_SPLINE_CURVE ( ( 0.9330127018922194093, 0.9330127018922198534, 1.000000000000000000, 0.8660254037844387076, 1.000000000000000000, 0.8660254037844387076, 1.000000000000000000, 0.9330127018922194093, 0.9330127018922194093 ) ) 
 REPRESENTATION_ITEM ( '' )  );
#9465=EDGE_CURVE ( 'NONE', #16189, #22108, #15273, .T. ) ;
#9469=CARTESIAN_POINT ( 'NONE',  ( 4.000000000000001776, 29.85624999877096997, 11.30940107675849760 ) ) ;
#9470=CARTESIAN_POINT ( 'NONE',  ( 3.756430356250002323, 28.81562499938548427, 11.16877607737301226 ) ) ;
#9477=CARTESIAN_POINT ( 'NONE',  ( 3.735045420075836212E-15, 25.70312499938548001, 4.662447845253954171 ) ) ;
#9494=CARTESIAN_POINT ( 'NONE',  ( 8.831537335106614961E-15, 26.63124999877096855, 12.99999999999999112 ) ) ;
#9499=CARTESIAN_POINT ( 'NONE',  ( 3.756430356250003655, 27.05312499938548498, 8.999999999999992895 ) ) ;
#9522=CARTESIAN_POINT ( 'NONE',  ( -3.756430356249996994, 26.82812499938548711, 8.999999999999992895 ) ) ;
#9523=CARTESIAN_POINT ( 'NONE',  ( 3.834746474454188013E-15, 28.26249999999999929, 4.999999999999992006 ) ) ;
#9528=DIRECTION ( 'NONE',  ( -0.000000000000000000, -1.000000000000000000, -0.000000000000000000 ) ) ;
#9562=ORIENTED_EDGE ( 'NONE', *, *, #23054, .T. ) ;
#9573=CARTESIAN_POINT ( 'NONE',  ( -3.999999999999997335, 26.61250000000000071, 11.30940107675849404 ) ) ;
#9589=ORIENTED_EDGE ( 'NONE', *, *, #22140, .T. ) ;
#9594=CARTESIAN_POINT ( 'NONE',  ( -3.756430356249995661, 27.24062499938548498, 6.831223922626973533 ) ) ;
#9596=ORIENTED_EDGE ( 'NONE', *, *, #13690, .F. ) ;
#9598=( BOUNDED_CURVE ( )  B_SPLINE_CURVE ( 2, ( #20978, #25017, #16658, #7106, #15220, #14706, #6975, #2925, #10632 ),
 .UNSPECIFIED., .F., .F. ) 
 B_SPLINE_CURVE_WITH_KNOTS ( ( 3, 2, 2, 2, 3 ),
 ( 0.3750000000000000000, 0.3833333333333333592, 0.4000000000000000222, 0.4166666666666666852, 0.4250000000000000444 ),
 .UNSPECIFIED. ) 
 CURVE ( )  GEOMETRIC_REPRESENTATION_ITEM ( )  RATIONAL_B_SPLINE_CURVE ( ( 0.9330127018922194093, 0.9330127018922194093, 1.000000000000000000, 0.8660254037844387076, 1.000000000000000000, 0.8660254037844387076, 1.000000000000000000, 0.9330127018922191873, 0.9330127018922194093 ) ) 
 REPRESENTATION_ITEM ( '' )  );
#9608=EDGE_CURVE ( 'NONE', #21413, #10718, #3787, .T. ) ;
#9617=CARTESIAN_POINT ( 'NONE',  ( 1.071796769724492338, 28.95759618943233704, 12.99999999999999467 ) ) ;
#9618=VECTOR ( 'NONE', #24407, 1000.000000000000000 ) ;
#9623=CARTESIAN_POINT ( 'NONE',  ( 1.878215178125004048, 29.26562499938548356, 5.746835883940462963 ) ) ;
#9630=CARTESIAN_POINT ( 'NONE',  ( -3.999999999999997335, 26.10624999877096997, 11.30940107675849404 ) ) ;
#9631=ADVANCED_FACE ( 'NONE', ( #10094 ), #1752, .T. ) ;
#9635=CARTESIAN_POINT ( 'NONE',  ( 3.735045420075836212E-15, 27.61562499938548498, 4.662447845253954171 ) ) ;
#9636=VECTOR ( 'NONE', #10157, 1000.000000000000000 ) ;
#9644=ADVANCED_FACE ( 'NONE', ( #9721 ), #17568, .T. ) ;
#9662=CARTESIAN_POINT ( 'NONE',  ( 1.878215178125004048, 27.12812499938548783, 5.746835883940462963 ) ) ;
#9674=VERTEX_POINT ( 'NONE', #3571 ) ;
#9689=CARTESIAN_POINT ( 'NONE',  ( 8.831537335106614961E-15, 27.53124999877097068, 12.99999999999999112 ) ) ;
#9694=DIRECTION ( 'NONE',  ( 0.8660254037844397068, -0.4999999999999983347, 0.000000000000000000 ) ) ;
#9700=CARTESIAN_POINT ( 'NONE',  ( 1.859271017917182139E-15, 29.78124999877096712, 12.99999999999999289 ) ) ;
#9701=CYLINDRICAL_SURFACE ( 'NONE', #2209, 4.000000000000000000 ) ;
#9703=CARTESIAN_POINT ( 'NONE',  ( -1.057460391440397258E-14, 28.71250000000000213, 4.999999999999992006 ) ) ;
#9704=ORIENTED_EDGE ( 'NONE', *, *, #13690, .T. ) ;
#9707=DIRECTION ( 'NONE',  ( -0.000000000000000000, -1.000000000000000000, -0.000000000000000000 ) ) ;
#9715=CARTESIAN_POINT ( 'NONE',  ( -1.999999999999998224, 27.10000000000000142, 12.46410161513774639 ) ) ;
#9716=CYLINDRICAL_SURFACE ( 'NONE', #25599, 5.500000000000000000 ) ;
#9721=FACE_OUTER_BOUND ( 'NONE', #381, .T. ) ;
#9737=ORIENTED_EDGE ( 'NONE', *, *, #1964, .F. ) ;
#9756=CARTESIAN_POINT ( 'NONE',  ( -1.878215178124998497, 29.49062499938548498, 12.25316411605951927 ) ) ;
#9761=CARTESIAN_POINT ( 'NONE',  ( -1.999999999999995781, 28.24374999877096570, 5.535898384862237620 ) ) ;
#9766=CARTESIAN_POINT ( 'NONE',  ( -3.756430356249996994, 29.07812499938548356, 8.999999999999992895 ) ) ;
#9781=CARTESIAN_POINT ( 'NONE',  ( 5.577813053751546416E-15, 25.73124999877097352, 12.99999999999999289 ) ) ;
#9787=CARTESIAN_POINT ( 'NONE',  ( -1.878215178124998497, 28.25312499938548427, 12.25316411605951927 ) ) ;
#9834=CARTESIAN_POINT ( 'NONE',  ( 3.752267015613588906E-15, 28.71250000000000568, 4.381197846482986158 ) ) ;
#9835=DIRECTION ( 'NONE',  ( -0.000000000000000000, -1.000000000000000000, -0.000000000000000000 ) ) ;
#9855=CARTESIAN_POINT ( 'NONE',  ( -3.756430356249997882, 29.11562499938548143, 11.16877607737301226 ) ) ;
#9856=CARTESIAN_POINT ( 'NONE',  ( 4.000000000000003553, 28.13124999877096855, 6.690598923241489970 ) ) ;
#9874=CARTESIAN_POINT ( 'NONE',  ( 4.000000000000001776, 29.40624999877096357, 11.30940107675849760 ) ) ;
#9879=CARTESIAN_POINT ( 'NONE',  ( 4.000000000000003553, 28.58124999877096784, 6.690598923241489970 ) ) ;
#9881=CARTESIAN_POINT ( 'NONE',  ( 4.000000000000003553, 29.50000000000000355, 8.999999999999992895 ) ) ;
#9883=CARTESIAN_POINT ( 'NONE',  ( -1.878215178124998497, 29.60312499938548569, 12.25316411605951927 ) ) ;
#9894=( BOUNDED_CURVE ( )  B_SPLINE_CURVE ( 2, ( #6701, #14436, #6320, #581, #22676 ),
 .UNSPECIFIED., .F., .F. ) 
 B_SPLINE_CURVE_WITH_KNOTS ( ( 3, 2, 3 ),
 ( 0.000000000000000000, 0.01666666666666666644, 0.02500000000000000486 ),
 .UNSPECIFIED. ) 
 CURVE ( )  GEOMETRIC_REPRESENTATION_ITEM ( )  RATIONAL_B_SPLINE_CURVE ( ( 1.000000000000000000, 0.8660254037844387076, 1.000000000000000000, 0.9330127018922194093, 0.9330127018922194093 ) ) 
 REPRESENTATION_ITEM ( '' )  );
#9906=CARTESIAN_POINT ( 'NONE',  ( 3.756430356250003655, 27.05312499938548498, 8.999999999999992895 ) ) ;
#9926=( LENGTH_UNIT ( ) NAMED_UNIT ( * ) SI_UNIT ( .MILLI., .METRE. ) );
#9946=ORIENTED_EDGE ( 'NONE', *, *, #3720, .F. ) ;
#9950=ORIENTED_EDGE ( 'NONE', *, *, #8784, .T. ) ;
#9953=DIRECTION ( 'NONE',  ( -0.000000000000000000, -1.000000000000000000, -0.000000000000000000 ) ) ;
#9955=CARTESIAN_POINT ( 'NONE',  ( -3.999999999999996003, 28.78750000000000142, 6.690598923241487306 ) ) ;
#9969=DIRECTION ( 'NONE',  ( 0.000000000000000000, 0.000000000000000000, 1.000000000000000000 ) ) ;
#9976=CARTESIAN_POINT ( 'NONE',  ( 2.000000000000000888, 29.81874999877096855, 12.46410161513774817 ) ) ;
#9981=VECTOR ( 'NONE', #8487, 1000.000000000000000 ) ;
#9985=CARTESIAN_POINT ( 'NONE',  ( -1.878215178124995832, 26.19062499938548427, 5.746835883940462963 ) ) ;
#9993=VECTOR ( 'NONE', #7749, 1000.000000000000000 ) ;
#10007=CARTESIAN_POINT ( 'NONE',  ( 2.000000000000000888, 27.11874999877096926, 12.46410161513774817 ) ) ;
#10011=CARTESIAN_POINT ( 'NONE',  ( -3.756430356249996994, 28.17812499938548498, 8.999999999999992895 ) ) ;
#10013=( BOUNDED_CURVE ( )  B_SPLINE_CURVE ( 2, ( #25580, #7665, #23615, #9874, #25830, #7915, #5694, #15901, #11960 ),
 .UNSPECIFIED., .F., .F. ) 
 B_SPLINE_CURVE_WITH_KNOTS ( ( 3, 2, 2, 2, 3 ),
 ( 0.8750000000000000000, 0.8833333333333333037, 0.9000000000000000222, 0.9166666666666666297, 0.9250000000000000444 ),
 .UNSPECIFIED. ) 
 CURVE ( )  GEOMETRIC_REPRESENTATION_ITEM ( )  RATIONAL_B_SPLINE_CURVE ( ( 0.9330127018922194093, 0.9330127018922194093, 1.000000000000000000, 0.8660254037844387076, 1.000000000000000000, 0.8660254037844387076, 1.000000000000000000, 0.9330127018922189652, 0.9330127018922194093 ) ) 
 REPRESENTATION_ITEM ( '' )  );
#10036=CARTESIAN_POINT ( 'NONE',  ( -3.756430356249997882, 28.21562499938548285, 11.16877607737301226 ) ) ;
#10043=CARTESIAN_POINT ( 'NONE',  ( 3.469446951953614189E-15, 40.00000000000000000, 8.999999999999992895 ) ) ;
#10055=AXIS2_PLACEMENT_3D ( 'NONE', #19027, #4905, #729 ) ;
#10059=FILL_AREA_STYLE_COLOUR ( '', #25618 ) ;
#10064=CARTESIAN_POINT ( 'NONE',  ( 4.000000000000003553, 29.50000000000000355, 8.999999999999992895 ) ) ;
#10065=CARTESIAN_POINT ( 'NONE',  ( 3.756430356250002323, 25.55312499938548498, 11.16877607737301403 ) ) ;
#10067=DIRECTION ( 'NONE',  ( 0.000000000000000000, 0.000000000000000000, -1.000000000000000000 ) ) ;
#10087=CARTESIAN_POINT ( 'NONE',  ( -3.999999999999996003, 29.23750000000000071, 6.690598923241487306 ) ) ;
#10094=FACE_OUTER_BOUND ( 'NONE', #18223, .T. ) ;
#10123=CARTESIAN_POINT ( 'NONE',  ( 1.878215178125000939, 26.86562499938548498, 12.25316411605952283 ) ) ;
#10137=CARTESIAN_POINT ( 'NONE',  ( 3.752267015613588906E-15, 28.65624999877096712, 4.381197846482986158 ) ) ;
#10141=CARTESIAN_POINT ( 'NONE',  ( 2.672651547586948120E-15, 28.29062499938548925, 13.33755215474603162 ) ) ;
#10154=AXIS2_PLACEMENT_3D ( 'NONE', #24797, #2569, #14737 ) ;
#10157=DIRECTION ( 'NONE',  ( -0.000000000000000000, -1.000000000000000000, -0.000000000000000000 ) ) ;
#10167=CARTESIAN_POINT ( 'NONE',  ( 1.878215178125004048, 25.66562499938548569, 5.746835883940462963 ) ) ;
#10191=CARTESIAN_POINT ( 'NONE',  ( 1.878215178125000939, 26.41562499938548214, 12.25316411605952283 ) ) ;
#10200=CARTESIAN_POINT ( 'NONE',  ( 4.000000000000001776, 28.56249999999999645, 11.30940107675849760 ) ) ;
#10205=ORIENTED_EDGE ( 'NONE', *, *, #25395, .F. ) ;
#10206=VERTEX_POINT ( 'NONE', #25094 ) ;
#10209=DIRECTION ( 'NONE',  ( -0.000000000000000000, -1.000000000000000000, -0.000000000000000000 ) ) ;
#10211=( BOUNDED_CURVE ( )  B_SPLINE_CURVE ( 2, ( #21621, #7505, #15878, #11685, #5674, #9856, #19407, #21892, #19660 ),
 .UNSPECIFIED., .F., .F. ) 
 B_SPLINE_CURVE_WITH_KNOTS ( ( 3, 2, 2, 2, 3 ),
 ( 0.5750000000000000666, 0.5833333333333333703, 0.5999999999999999778, 0.6166666666666666963, 0.6250000000000000000 ),
 .UNSPECIFIED. ) 
 CURVE ( )  GEOMETRIC_REPRESENTATION_ITEM ( )  RATIONAL_B_SPLINE_CURVE ( ( 0.9330127018922194093, 0.9330127018922198534, 1.000000000000000000, 0.8660254037844387076, 1.000000000000000000, 0.8660254037844387076, 1.000000000000000000, 0.9330127018922194093, 0.9330127018922194093 ) ) 
 REPRESENTATION_ITEM ( '' )  );
#10222=CARTESIAN_POINT ( 'NONE',  ( 1.859271017917182139E-15, 28.93749999999999645, 12.99999999999999289 ) ) ;
#10223=CARTESIAN_POINT ( 'NONE',  ( 3.469446951953614189E-15, 25.00000000000000000, 8.999999999999992895 ) ) ;
#10238=CARTESIAN_POINT ( 'NONE',  ( -1.878215178124998497, 27.24062499938548498, 12.25316411605951927 ) ) ;
#10240=EDGE_CURVE ( 'NONE', #18460, #5942, #15169, .T. ) ;
#10257=CARTESIAN_POINT ( 'NONE',  ( 4.000000000000001776, 28.05624999877096926, 11.30940107675849760 ) ) ;
#10274=CARTESIAN_POINT ( 'NONE',  ( 1.859271017917182139E-15, 29.33124999877096428, 12.99999999999999289 ) ) ;
#10279=CARTESIAN_POINT ( 'NONE',  ( 3.834746474454188013E-15, 25.56250000000000000, 4.999999999999992006 ) ) ;
#10286=CARTESIAN_POINT ( 'NONE',  ( 1.878215178125004048, 29.37812499938548783, 5.746835883940462963 ) ) ;
#10302=CARTESIAN_POINT ( 'NONE',  ( -3.137519842735244810E-15, 26.85624999877096641, 4.999999999999991118 ) ) ;
#10310=CARTESIAN_POINT ( 'NONE',  ( 3.756430356250003655, 27.39062499938548356, 8.999999999999992895 ) ) ;
#10331=CARTESIAN_POINT ( 'NONE',  ( -3.999999999999996447, 28.82499999999999929, 8.999999999999992895 ) ) ;
#10358=CARTESIAN_POINT ( 'NONE',  ( -1.878215178124998497, 26.79062499938548214, 12.25316411605951927 ) ) ;
#10377=CARTESIAN_POINT ( 'NONE',  ( 3.752267015613588906E-15, 29.10624999877096997, 4.381197846482986158 ) ) ;
#10399=DIRECTION ( 'NONE',  ( 0.000000000000000000, 0.000000000000000000, -1.000000000000000000 ) ) ;
#10408=CARTESIAN_POINT ( 'NONE',  ( 2.672651547586948120E-15, 25.47812499938548569, 13.33755215474602984 ) ) ;
#10412=AXIS2_PLACEMENT_3D ( 'NONE', #23883, #15773, #19436 ) ;
#10445=CARTESIAN_POINT ( 'NONE',  ( 3.756430356250002323, 26.00312499938548427, 11.16877607737301403 ) ) ;
#10483=CARTESIAN_POINT ( 'NONE',  ( 3.878215178125003604, 29.82343749907822783, 8.999999999999992895 ) ) ;
#10500=CARTESIAN_POINT ( 'NONE',  ( -3.999999999999995559, 29.18124999877096926, 6.690598923241487306 ) ) ;
#10502=CARTESIAN_POINT ( 'NONE',  ( 1.071796769724498999, 28.45134618820330275, 12.99999999999998757 ) ) ;
#10503=CARTESIAN_POINT ( 'NONE',  ( 3.756430356250002323, 27.35312499938547859, 11.16877607737301226 ) ) ;
#10514=CARTESIAN_POINT ( 'NONE',  ( -3.999999999999996447, 26.12500000000000355, 8.999999999999992895 ) ) ;
#10523=CARTESIAN_POINT ( 'NONE',  ( 4.000000000000001776, 29.85624999877096997, 11.30940107675849760 ) ) ;
#10547=CARTESIAN_POINT ( 'NONE',  ( 3.834746474454188013E-15, 27.81249999999999645, 4.999999999999992006 ) ) ;
#10549=CARTESIAN_POINT ( 'NONE',  ( -3.756430356249997882, 29.11562499938548143, 11.16877607737301226 ) ) ;
#10578=CARTESIAN_POINT ( 'NONE',  ( 1.878215178125004048, 25.21562499938548285, 5.746835883940462963 ) ) ;
#10618=EDGE_CURVE ( 'NONE', #4929, #3732, #11569, .T. ) ;
#10621=EDGE_CURVE ( 'NONE', #10854, #14526, #16260, .T. ) ;
#10631=CARTESIAN_POINT ( 'NONE',  ( 2.620986760973688460E-15, 25.33750000000000568, 13.61880215351699874 ) ) ;
#10632=CARTESIAN_POINT ( 'NONE',  ( -3.137519842735244810E-15, 27.30624999877096926, 4.999999999999991118 ) ) ;
#10646=CARTESIAN_POINT ( 'NONE',  ( -3.756430356249996994, 26.37812499938548783, 8.999999999999992895 ) ) ;
#10672=CARTESIAN_POINT ( 'NONE',  ( 1.878215178125004048, 28.92812499938548854, 5.746835883940462963 ) ) ;
#10701=CARTESIAN_POINT ( 'NONE',  ( 1.878215178125000939, 28.66562499938548569, 12.25316411605952283 ) ) ;
#10718=VERTEX_POINT ( 'NONE', #7085 ) ;
#10753=CARTESIAN_POINT ( 'NONE',  ( -1.878215178124995832, 29.34062499938548285, 5.746835883940462963 ) ) ;
#10770=CARTESIAN_POINT ( 'NONE',  ( -3.756430356249995661, 25.89062499938548356, 6.831223922626973533 ) ) ;
#10799=CARTESIAN_POINT ( 'NONE',  ( 2.000000000000003997, 27.77500000000000213, 5.535898384862238508 ) ) ;
#10801=CARTESIAN_POINT ( 'NONE',  ( 3.756430356250002323, 26.90312499938548640, 11.16877607737301226 ) ) ;
#10831=CARTESIAN_POINT ( 'NONE',  ( 3.735045420075836212E-15, 27.95312499938548001, 4.662447845253954171 ) ) ;
#10854=VERTEX_POINT ( 'NONE', #3635 ) ;
#10861=VECTOR ( 'NONE', #9289, 1000.000000000000000 ) ;
#10879=VERTEX_POINT ( 'NONE', #23769 ) ;
#10884=CARTESIAN_POINT ( 'NONE',  ( -1.878215178124995832, 28.44062499938548427, 5.746835883940462963 ) ) ;
#10888=CARTESIAN_POINT ( 'NONE',  ( 2.000000000000000888, 26.27499999999999858, 12.46410161513774817 ) ) ;
#10907=CARTESIAN_POINT ( 'NONE',  ( 2.000000000000000888, 28.91874999877096997, 12.46410161513774817 ) ) ;
#10937=CARTESIAN_POINT ( 'NONE',  ( 1.071796769724494558, 27.79240381056766651, 4.999999999999992895 ) ) ;
#10939=CARTESIAN_POINT ( 'NONE',  ( 3.735045420075836212E-15, 28.85312499938548569, 4.662447845253954171 ) ) ;
#10979=CARTESIAN_POINT ( 'NONE',  ( -1.999999999999995781, 29.59374999877096712, 5.535898384862237620 ) ) ;
#10991=ORIENTED_EDGE ( 'NONE', *, *, #714, .T. ) ;
#11013=CARTESIAN_POINT ( 'NONE',  ( -1.999999999999995781, 25.60000000000000142, 5.535898384862237620 ) ) ;
#11026=CARTESIAN_POINT ( 'NONE',  ( 3.756430356250002323, 29.15312499938548640, 11.16877607737301226 ) ) ;
#11040=CARTESIAN_POINT ( 'NONE',  ( 1.878215178125004048, 27.12812499938548783, 5.746835883940462963 ) ) ;
#11056=( BOUNDED_CURVE ( )  B_SPLINE_CURVE ( 2, ( #16442, #2423, #6357, #18148, #14209, #220, #22310, #16168, #20332 ),
 .UNSPECIFIED., .F., .F. ) 
 B_SPLINE_CURVE_WITH_KNOTS ( ( 3, 2, 2, 2, 3 ),
 ( 0.5250000000000000222, 0.5333333333333333259, 0.5500000000000000444, 0.5666666666666666519, 0.5750000000000000666 ),
 .UNSPECIFIED. ) 
 CURVE ( )  GEOMETRIC_REPRESENTATION_ITEM ( )  RATIONAL_B_SPLINE_CURVE ( ( 0.9330127018922194093, 0.9330127018922194093, 1.000000000000000000, 0.8660254037844387076, 1.000000000000000000, 0.8660254037844387076, 1.000000000000000000, 0.9330127018922189652, 0.9330127018922194093 ) ) 
 REPRESENTATION_ITEM ( '' )  );
#11067=CARTESIAN_POINT ( 'NONE',  ( 1.878215178125000939, 27.31562499938548427, 12.25316411605952283 ) ) ;
#11077=CARTESIAN_POINT ( 'NONE',  ( -3.756430356249997438, 25.51562499938548356, 11.16877607737301048 ) ) ;
#11096=CARTESIAN_POINT ( 'NONE',  ( -3.756430356249996994, 28.06562499938548427, 8.999999999999992895 ) ) ;
#11103=CARTESIAN_POINT ( 'NONE',  ( 1.071796769724495668, 27.55134618820330061, 12.99999999999999112 ) ) ;
#11143=CARTESIAN_POINT ( 'NONE',  ( 4.000000000000003553, 25.90000000000000213, 8.999999999999992895 ) ) ;
#11145=CARTESIAN_POINT ( 'NONE',  ( -1.071796769724488563, 26.66740381056766651, 12.99999999999999289 ) ) ;
#11149=CARTESIAN_POINT ( 'NONE',  ( 1.859271017917182139E-15, 28.48749999999999716, 12.99999999999999289 ) ) ;
#11160=CARTESIAN_POINT ( 'NONE',  ( 3.756430356250003655, 27.05312499938548498, 8.999999999999992895 ) ) ;
#11163=ORIENTED_EDGE ( 'NONE', *, *, #24238, .T. ) ;
#11184=CARTESIAN_POINT ( 'NONE',  ( -3.756430356249996994, 27.16562499938548214, 8.999999999999992895 ) ) ;
#11196=CARTESIAN_POINT ( 'NONE',  ( 3.735045420075836212E-15, 25.36562499938548854, 4.662447845253954171 ) ) ;
#11214=CARTESIAN_POINT ( 'NONE',  ( -1.878215178124998497, 28.14062499938548356, 12.25316411605951927 ) ) ;
#11220=CARTESIAN_POINT ( 'NONE',  ( -3.756430356249996994, 25.92812499938548498, 8.999999999999992895 ) ) ;
#11232=VECTOR ( 'NONE', #4651, 1000.000000000000000 ) ;
#11271=CARTESIAN_POINT ( 'NONE',  ( -3.999999999999996447, 26.57500000000000284, 8.999999999999992895 ) ) ;
#11288=EDGE_LOOP ( 'NONE', ( #17365, #18352, #9185, #20759, #2640, #13627, #13677, #8451, #5002, #13247, #11620, #13539, #8316, #6085, #25246, #19697, #13716, #4198, #15684, #19400, #25302, #6905, #13710, #16681 ) ) ;
#11295=CARTESIAN_POINT ( 'NONE',  ( 1.878215178125004048, 28.47812499938548569, 5.746835883940462963 ) ) ;
#11307=CARTESIAN_POINT ( 'NONE',  ( 1.878215178125000939, 25.51562499938548356, 12.25316411605952283 ) ) ;
#11316=VECTOR ( 'NONE', #23383, 999.9999999999998863 ) ;
#11323=CARTESIAN_POINT ( 'NONE',  ( -1.878215178124998497, 28.59062499938548285, 12.25316411605951927 ) ) ;
#11329=CARTESIAN_POINT ( 'NONE',  ( 2.000000000000003997, 26.81874999877096855, 5.535898384862238508 ) ) ;
#11334=CARTESIAN_POINT ( 'NONE',  ( 3.756430356250003655, 25.70312499938548356, 8.999999999999992895 ) ) ;
#11341=AXIS2_PLACEMENT_3D ( 'NONE', #21443, #1559, #12848 ) ;
#11371=VECTOR ( 'NONE', #22835, 1000.000000000000000 ) ;
#11413=CARTESIAN_POINT ( 'NONE',  ( -1.999999999999995781, 26.50000000000000355, 5.535898384862237620 ) ) ;
#11414=DIRECTION ( 'NONE',  ( -0.000000000000000000, -1.000000000000000000, -0.000000000000000000 ) ) ;
#11431=ORIENTED_EDGE ( 'NONE', *, *, #22170, .F. ) ;
#11433=CARTESIAN_POINT ( 'NONE',  ( -3.756430356249997882, 28.21562499938548285, 11.16877607737301226 ) ) ;
#11441=CARTESIAN_POINT ( 'NONE',  ( -1.878215178124998497, 25.44062499938548427, 12.25316411605951927 ) ) ;
#11456=CARTESIAN_POINT ( 'NONE',  ( 4.000000000000003553, 28.18750000000000000, 6.690598923241489970 ) ) ;
#11461=CARTESIAN_POINT ( 'NONE',  ( 3.752267015613588906E-15, 25.50624999877097565, 4.381197846482986158 ) ) ;
#11464=CARTESIAN_POINT ( 'NONE',  ( 4.000000000000001776, 29.46250000000000213, 11.30940107675849760 ) ) ;
#11467=CARTESIAN_POINT ( 'NONE',  ( 2.672651547586948120E-15, 25.59062499938548640, 13.33755215474603162 ) ) ;
#11468=EDGE_CURVE ( 'NONE', #23620, #408, #16039, .T. ) ;
#11489=CARTESIAN_POINT ( 'NONE',  ( 1.878215178125000939, 26.97812499938548569, 12.25316411605952283 ) ) ;
#11523=CARTESIAN_POINT ( 'NONE',  ( -3.999999999999996447, 25.67500000000000071, 8.999999999999992895 ) ) ;
#11536=CARTESIAN_POINT ( 'NONE',  ( -3.999999999999997335, 27.06250000000000000, 11.30940107675849404 ) ) ;
#11552=CARTESIAN_POINT ( 'NONE',  ( 3.756430356250003655, 28.40312499938548640, 8.999999999999992895 ) ) ;
#11554=ORIENTED_EDGE ( 'NONE', *, *, #8385, .F. ) ;
#11569=LINE ( 'NONE', #10483, #20089 ) ;
#11575=CYLINDRICAL_SURFACE ( 'NONE', #21147, 4.000000000000000000 ) ;
#11579=CARTESIAN_POINT ( 'NONE',  ( 3.752267015613588906E-15, 25.95624999877096784, 4.381197846482986158 ) ) ;
#11583=CARTESIAN_POINT ( 'NONE',  ( -3.756430356249996994, 25.47812499938548569, 8.999999999999992895 ) ) ;
#11589=EDGE_CURVE ( 'NONE', #13240, #1665, #910, .T. ) ;
#11608=CARTESIAN_POINT ( 'NONE',  ( 2.672651547586948120E-15, 28.74062499938548498, 13.33755215474602984 ) ) ;
#11612=ORIENTED_EDGE ( 'NONE', *, *, #3705, .T. ) ;
#11618=AXIS2_PLACEMENT_3D ( 'NONE', #6926, #20787, #17271 ) ;
#11620=ORIENTED_EDGE ( 'NONE', *, *, #20025, .T. ) ;
#11622=EDGE_CURVE ( 'NONE', #16822, #19025, #13334, .T. ) ;
#11633=ADVANCED_FACE ( 'NONE', ( #7438 ), #17652, .F. ) ;
#11655=ORIENTED_EDGE ( 'NONE', *, *, #24388, .F. ) ;
#11660=CARTESIAN_POINT ( 'NONE',  ( 2.000000000000003997, 26.42500000000000071, 5.535898384862238508 ) ) ;
#11674=CARTESIAN_POINT ( 'NONE',  ( -1.071796769724488563, 29.36740381056767291, 12.99999999999999289 ) ) ;
#11685=CARTESIAN_POINT ( 'NONE',  ( 4.000000000000001776, 28.05624999877096570, 11.30940107675849760 ) ) ;
#11715=CARTESIAN_POINT ( 'NONE',  ( 3.959305671612554781E-15, 25.00000000000000000, 12.99999999999999289 ) ) ;
#11717=CARTESIAN_POINT ( 'NONE',  ( 2.000000000000003997, 26.36874999877096926, 5.535898384862238508 ) ) ;
#11721=CARTESIAN_POINT ( 'NONE',  ( 3.756430356250003655, 29.30312499938548498, 8.999999999999992895 ) ) ;
#11726=VERTEX_POINT ( 'NONE', #5999 ) ;
#11746=CARTESIAN_POINT ( 'NONE',  ( 2.672651547586948120E-15, 26.94062499938548783, 13.33755215474602984 ) ) ;
#11764=CYLINDRICAL_SURFACE ( 'NONE', #8033, 4.000000000000000000 ) ;
#11794=ORIENTED_EDGE ( 'NONE', *, *, #7727, .F. ) ;
#11801=CARTESIAN_POINT ( 'NONE',  ( -3.999999999999996447, 26.12500000000000355, 8.999999999999992895 ) ) ;
#11818=EDGE_CURVE ( 'NONE', #19820, #10854, #14288, .T. ) ;
#11820=CARTESIAN_POINT ( 'NONE',  ( -3.999999999999997335, 26.10624999877096997, 11.30940107675849404 ) ) ;
#11825=VERTEX_POINT ( 'NONE', #2716 ) ;
#11846=CARTESIAN_POINT ( 'NONE',  ( 2.000000000000003997, 27.71874999877097068, 5.535898384862238508 ) ) ;
#11850=CARTESIAN_POINT ( 'NONE',  ( -3.756430356249997438, 29.56562499938549493, 11.16877607737301048 ) ) ;
#11875=CARTESIAN_POINT ( 'NONE',  ( 3.756430356250004099, 27.09062499938548285, 6.831223922626973533 ) ) ;
#11909=CARTESIAN_POINT ( 'NONE',  ( 3.469446951953614189E-15, 46.00000000000000000, 8.999999999999992895 ) ) ;
#11919=CARTESIAN_POINT ( 'NONE',  ( 4.000000000000001776, 28.56249999999999645, 11.30940107675849760 ) ) ;
#11937=CARTESIAN_POINT ( 'NONE',  ( 1.859271017917182139E-15, 26.18124999877096570, 12.99999999999999289 ) ) ;
#11939=CARTESIAN_POINT ( 'NONE',  ( -3.756430356249995661, 29.04062499938548569, 6.831223922626973533 ) ) ;
#11946=CARTESIAN_POINT ( 'NONE',  ( 1.878215178125004048, 26.11562499938548498, 5.746835883940462963 ) ) ;
#11947=DIRECTION ( 'NONE',  ( 0.000000000000000000, 1.000000000000000000, 0.000000000000000000 ) ) ;
#11960=CARTESIAN_POINT ( 'NONE',  ( -1.057460391440397258E-14, 29.55624999877096926, 4.999999999999992006 ) ) ;
#11964=CARTESIAN_POINT ( 'NONE',  ( 4.000000000000003553, 27.64374999877096784, 8.999999999999992895 ) ) ;
#11968=CARTESIAN_POINT ( 'NONE',  ( -3.756430356249996105, 27.69062499938548072, 6.831223922626973533 ) ) ;
#11990=CARTESIAN_POINT ( 'NONE',  ( 3.756430356250003655, 27.50312499938548427, 8.999999999999992895 ) ) ;
#11992=FACE_OUTER_BOUND ( 'NONE', #12821, .T. ) ;
#12015=CARTESIAN_POINT ( 'NONE',  ( -3.756430356249996994, 27.16562499938548214, 8.999999999999992895 ) ) ;
#12027=EDGE_CURVE ( 'NONE', #12396, #1940, #19604, .T. ) ;
#12035=ORIENTED_EDGE ( 'NONE', *, *, #25301, .F. ) ;
#12040=CARTESIAN_POINT ( 'NONE',  ( 3.469446951953614189E-15, 40.00000000000000000, 4.999999999999992006 ) ) ;
#12057=ADVANCED_FACE ( 'NONE', ( #17240 ), #20766, .T. ) ;
#12076=CARTESIAN_POINT ( 'NONE',  ( 3.735045420075836212E-15, 26.60312499938547859, 4.662447845253954171 ) ) ;
#12098=CARTESIAN_POINT ( 'NONE',  ( 4.000000000000003553, 27.68124999877096926, 6.690598923241489970 ) ) ;
#12102=CARTESIAN_POINT ( 'NONE',  ( 3.735045420075836212E-15, 28.96562499938548640, 4.662447845253954171 ) ) ;
#12115=CARTESIAN_POINT ( 'NONE',  ( -3.999999999999995559, 27.38124999877096855, 6.690598923241487306 ) ) ;
#12128=CARTESIAN_POINT ( 'NONE',  ( 3.756430356250003655, 25.59062499938548285, 8.999999999999992895 ) ) ;
#12157=CARTESIAN_POINT ( 'NONE',  ( -1.878215178124998497, 26.79062499938548214, 12.25316411605951927 ) ) ;
#12163=CARTESIAN_POINT ( 'NONE',  ( -3.999999999999997335, 27.96250000000000213, 11.30940107675849404 ) ) ;
#12181=CARTESIAN_POINT ( 'NONE',  ( 4.000000000000003553, 29.50000000000000355, 8.999999999999992895 ) ) ;
#12204=VECTOR ( 'NONE', #4959, 1000.000000000000000 ) ;
#12215=CARTESIAN_POINT ( 'NONE',  ( 2.672651547586948120E-15, 26.82812499938548356, 13.33755215474602984 ) ) ;
#12233=CARTESIAN_POINT ( 'NONE',  ( 2.000000000000003997, 27.26874999877097139, 5.535898384862238508 ) ) ;
#12236=ORIENTED_EDGE ( 'NONE', *, *, #22026, .F. ) ;
#12238=CARTESIAN_POINT ( 'NONE',  ( 1.878215178125004048, 28.47812499938548569, 5.746835883940462963 ) ) ;
#12245=CARTESIAN_POINT ( 'NONE',  ( 1.626862140677534194E-14, 27.98124999877096997, 12.99999999999999289 ) ) ;
#12262=CARTESIAN_POINT ( 'NONE',  ( -1.878215178124998497, 29.15312499938548640, 12.25316411605951927 ) ) ;
#12273=ORIENTED_EDGE ( 'NONE', *, *, #20173, .T. ) ;
#12289=DIRECTION ( 'NONE',  ( 1.000000000000000000, 0.000000000000000000, -0.000000000000000000 ) ) ;
#12291=CARTESIAN_POINT ( 'NONE',  ( -1.878215178124995832, 26.19062499938548427, 5.746835883940462963 ) ) ;
#12336=EDGE_CURVE ( 'NONE', #12422, #2907, #269, .T. ) ;
#12343=CARTESIAN_POINT ( 'NONE',  ( -3.756430356249996994, 27.16562499938548214, 8.999999999999992895 ) ) ;
#12351=CARTESIAN_POINT ( 'NONE',  ( 3.834746474454188013E-15, 26.01249999999999574, 4.999999999999992006 ) ) ;
#12358=ORIENTED_EDGE ( 'NONE', *, *, #3927, .F. ) ;
#12359=CARTESIAN_POINT ( 'NONE',  ( 3.752267015613588906E-15, 27.75624999877096855, 4.381197846482986158 ) ) ;
#12385=CARTESIAN_POINT ( 'NONE',  ( -1.878215178124998497, 26.34062499938548285, 12.25316411605951927 ) ) ;
#12395=CARTESIAN_POINT ( 'NONE',  ( 3.469446951953614189E-15, 40.00000000000000000, 8.999999999999992895 ) ) ;
#12396=VERTEX_POINT ( 'NONE', #14000 ) ;
#12406=( NAMED_UNIT ( * ) PLANE_ANGLE_UNIT ( ) SI_UNIT ( $, .RADIAN. ) );
#12410=CARTESIAN_POINT ( 'NONE',  ( 1.878215178125000939, 25.96562499938548285, 12.25316411605952283 ) ) ;
#12419=ORIENTED_EDGE ( 'NONE', *, *, #10240, .F. ) ;
#12422=VERTEX_POINT ( 'NONE', #10064 ) ;
#12463=CARTESIAN_POINT ( 'NONE',  ( -3.756430356249997882, 26.75312499938548427, 11.16877607737301226 ) ) ;
#12481=CARTESIAN_POINT ( 'NONE',  ( 1.878215178125004048, 25.77812499938548640, 5.746835883940462963 ) ) ;
#12513=CARTESIAN_POINT ( 'NONE',  ( 3.735045420075836212E-15, 29.41562499938548569, 4.662447845253954171 ) ) ;
#12520=CARTESIAN_POINT ( 'NONE',  ( -1.999999999999995781, 28.75000000000000000, 5.535898384862237620 ) ) ;
#12525=CARTESIAN_POINT ( 'NONE',  ( 3.469446951953614189E-15, 40.00000000000000000, 4.999999999999992006 ) ) ;
#12545=CARTESIAN_POINT ( 'NONE',  ( 3.735045420075836212E-15, 26.60312499938547859, 4.662447845253954171 ) ) ;
#12561=EDGE_LOOP ( 'NONE', ( #2452, #966, #20642, #6255 ) ) ;
#12606=CARTESIAN_POINT ( 'NONE',  ( -3.999999999999996003, 25.18750000000000000, 6.690598923241487306 ) ) ;
#12628=CARTESIAN_POINT ( 'NONE',  ( 2.620986760973688460E-15, 29.78124999877096712, 13.61880215351699874 ) ) ;
#12643=FACE_OUTER_BOUND ( 'NONE', #2528, .T. ) ;
#12655=CARTESIAN_POINT ( 'NONE',  ( -3.756430356249995661, 29.04062499938548569, 6.831223922626973533 ) ) ;
#12658=EDGE_LOOP ( 'NONE', ( #7864, #16199, #21591, #9029 ) ) ;
#12687=CARTESIAN_POINT ( 'NONE',  ( -3.756430356249996994, 27.61562499938548143, 8.999999999999992895 ) ) ;
#12705=ORIENTED_EDGE ( 'NONE', *, *, #2692, .F. ) ;
#12708=( BOUNDED_CURVE ( )  B_SPLINE_CURVE ( 2, ( #5359, #25366, #23159, #10500, #3401, #22538, #13219, #23408, #3263 ),
 .UNSPECIFIED., .F., .F. ) 
 B_SPLINE_CURVE_WITH_KNOTS ( ( 3, 2, 2, 2, 3 ),
 ( 0.8250000000000000666, 0.8333333333333333703, 0.8499999999999999778, 0.8666666666666666963, 0.8750000000000000000 ),
 .UNSPECIFIED. ) 
 CURVE ( )  GEOMETRIC_REPRESENTATION_ITEM ( )  RATIONAL_B_SPLINE_CURVE ( ( 0.9330127018922194093, 0.9330127018922198534, 1.000000000000000000, 0.8660254037844387076, 1.000000000000000000, 0.8660254037844387076, 1.000000000000000000, 0.9330127018922194093, 0.9330127018922194093 ) ) 
 REPRESENTATION_ITEM ( '' )  );
#12710=ORIENTED_EDGE ( 'NONE', *, *, #5202, .F. ) ;
#12739=CARTESIAN_POINT ( 'NONE',  ( 4.000000000000003553, 25.93750000000000000, 6.690598923241489970 ) ) ;
#12742=DIRECTION ( 'NONE',  ( 0.000000000000000000, 0.000000000000000000, -1.000000000000000000 ) ) ;
#12756=CARTESIAN_POINT ( 'NONE',  ( 3.756430356250002323, 26.56562499938548427, 11.16877607737301226 ) ) ;
#12783=CARTESIAN_POINT ( 'NONE',  ( -1.878215178124995832, 27.54062499938548214, 5.746835883940462963 ) ) ;
#12793=LINE ( 'NONE', #12525, #9981 ) ;
#12794=VERTEX_POINT ( 'NONE', #10274 ) ;
#12812=CARTESIAN_POINT ( 'NONE',  ( 3.469446951953614189E-15, 34.00000000000000000, 8.999999999999992895 ) ) ;
#12814=CARTESIAN_POINT ( 'NONE',  ( 1.878215178125000939, 25.62812499938548783, 12.25316411605952283 ) ) ;
#12821=EDGE_LOOP ( 'NONE', ( #23891, #9704 ) ) ;
#12848=DIRECTION ( 'NONE',  ( 0.000000000000000000, -0.000000000000000000, 1.000000000000000000 ) ) ;
#12849=ORIENTED_EDGE ( 'NONE', *, *, #8035, .T. ) ;
#12851=ORIENTED_EDGE ( 'NONE', *, *, #2692, .T. ) ;
#12856=CARTESIAN_POINT ( 'NONE',  ( -1.999999999999998224, 25.30000000000000426, 12.46410161513774639 ) ) ;
#12857=CARTESIAN_POINT ( 'NONE',  ( -1.071796769724481901, 28.41115380933862866, 12.99999999999999645 ) ) ;
#12862=CARTESIAN_POINT ( 'NONE',  ( -3.999999999999996447, 28.37500000000000000, 8.999999999999992895 ) ) ;
#12876=CARTESIAN_POINT ( 'NONE',  ( -1.878215178124995832, 25.85312499938548569, 5.746835883940462963 ) ) ;
#12887=CARTESIAN_POINT ( 'NONE',  ( 3.959305671612554781E-15, 40.00000000000000000, 12.99999999999999289 ) ) ;
#12890=( BOUNDED_CURVE ( )  B_SPLINE_CURVE ( 2, ( #16005, #21612, #23972, #6053, #23701, #25797, #15616, #11674, #19650 ),
 .UNSPECIFIED., .F., .F. ) 
 B_SPLINE_CURVE_WITH_KNOTS ( ( 3, 2, 2, 2, 3 ),
 ( 0.9250000000000000444, 0.9333333333333333481, 0.9499999999999999556, 0.9666666666666666741, 0.9749999999999999778 ),
 .UNSPECIFIED. ) 
 CURVE ( )  GEOMETRIC_REPRESENTATION_ITEM ( )  RATIONAL_B_SPLINE_CURVE ( ( 0.9330127018922194093, 0.9330127018922198534, 1.000000000000000000, 0.8660254037844387076, 1.000000000000000000, 0.8660254037844387076, 1.000000000000000000, 0.9330127018922194093, 0.9330127018922194093 ) ) 
 REPRESENTATION_ITEM ( '' )  );
#12908=CARTESIAN_POINT ( 'NONE',  ( 1.878215178125004048, 28.36562499938548143, 5.746835883940462963 ) ) ;
#12937=CARTESIAN_POINT ( 'NONE',  ( 3.735045420075836212E-15, 29.30312499938548498, 4.662447845253954171 ) ) ;
#12943=CARTESIAN_POINT ( 'NONE',  ( 1.878215178125004048, 26.22812499938548569, 5.746835883940462963 ) ) ;
#12946=CARTESIAN_POINT ( 'NONE',  ( -1.057460391440397258E-14, 29.55624999877096926, 4.999999999999992006 ) ) ;
#12957=ORIENTED_EDGE ( 'NONE', *, *, #3693, .T. ) ;
#12974=CARTESIAN_POINT ( 'NONE',  ( -1.057460391440397258E-14, 29.16249999999999787, 4.999999999999992006 ) ) ;
#12975=( BOUNDED_CURVE ( )  B_SPLINE_CURVE ( 2, ( #18072, #4186, #16366, #14651, #24332, #12163, #2484, #14400, #20384 ),
 .UNSPECIFIED., .F., .F. ) 
 B_SPLINE_CURVE_WITH_KNOTS ( ( 3, 2, 2, 2, 3 ),
 ( 0.6250000000000000000, 0.6333333333333333037, 0.6500000000000000222, 0.6666666666666666297, 0.6750000000000000444 ),
 .UNSPECIFIED. ) 
 CURVE ( )  GEOMETRIC_REPRESENTATION_ITEM ( )  RATIONAL_B_SPLINE_CURVE ( ( 0.9330127018922194093, 0.9330127018922194093, 1.000000000000000000, 0.8660254037844387076, 1.000000000000000000, 0.8660254037844387076, 1.000000000000000000, 0.9330127018922189652, 0.9330127018922194093 ) ) 
 REPRESENTATION_ITEM ( '' )  );
#12986=ADVANCED_FACE ( 'NONE', ( #6883 ), #4799, .T. ) ;
#12997=CARTESIAN_POINT ( 'NONE',  ( 4.000000000000001776, 25.41250000000000142, 11.30940107675849760 ) ) ;
#13000=CARTESIAN_POINT ( 'NONE',  ( 4.000000000000003553, 26.35000000000000142, 8.999999999999992895 ) ) ;
#13008=EDGE_LOOP ( 'NONE', ( #8736, #5898, #21116, #481 ) ) ;
#13014=CARTESIAN_POINT ( 'NONE',  ( -3.999999999999996447, 27.02500000000000213, 8.999999999999992895 ) ) ;
#13016=CARTESIAN_POINT ( 'NONE',  ( 3.735045420075836212E-15, 25.81562499938548783, 4.662447845253954171 ) ) ;
#13033=VECTOR ( 'NONE', #21845, 999.9999999999998863 ) ;
#13044=CARTESIAN_POINT ( 'NONE',  ( 3.756430356250003655, 28.74062499938548498, 8.999999999999992895 ) ) ;
#13056=CARTESIAN_POINT ( 'NONE',  ( -3.756430356249996105, 27.24062499938548498, 6.831223922626973533 ) ) ;
#13075=CARTESIAN_POINT ( 'NONE',  ( -3.756430356249997438, 28.55312499938548498, 11.16877607737301048 ) ) ;
#13081=CARTESIAN_POINT ( 'NONE',  ( -3.756430356249995661, 25.89062499938548356, 6.831223922626973533 ) ) ;
#13082=CARTESIAN_POINT ( 'NONE',  ( 1.071796769724494558, 27.73615380933863861, 4.999999999999992895 ) ) ;
#13088=DIRECTION ( 'NONE',  ( 0.000000000000000000, 0.000000000000000000, -1.000000000000000000 ) ) ;
#13129=CARTESIAN_POINT ( 'NONE',  ( 3.756430356250004099, 28.77812499938548285, 6.831223922626973533 ) ) ;
#13130=CARTESIAN_POINT ( 'NONE',  ( 3.834746474454188013E-15, 28.20624999877096428, 4.999999999999992006 ) ) ;
#13135=( BOUNDED_CURVE ( )  B_SPLINE_CURVE ( 2, ( #2618, #2097, #10578, #2475, #6141, #2234, #2354, #14265, #20377, #22232, #8507, #10065, #14511, #18574, #24450, #16488, #4315, #397, #271, #22482, #15972, #6405, #12410, #10445, #23937, #22353, #4564, #8366, #12291, #18440, #6528, #148, #535, #14395, #10191, #4179, #18187, #6020, #8239, #12545, #22090, #20523, #20257, #19992, #12157, #20132, #7984, #16215, #14125, #4437, #8119, #24058, #14001, #21972, #12015, #24185, #4047, #6274, #16094, #16357, #10310, #18304, #24325, #5218, #16996, #23139, #12687, #22755, #24843, #14644, #20657, #6656, #20917, #13196, #16740, #10831, #14903, #15170, #11096, #20781, #11214, #21168, #16878, #3240, #2739, #657, #21051, #24708, #2862, #3001, #6919, #13075, #22874, #1154, #10701, #7182, #8626, #17124, #9132, #4956, #18955, #22626, #8896, #18687, #24961, #5096, #3128, #16604, #15031, #24567, #1042, #12937, #19073, #25096, #775, #4714, #7044, #18825, #4832, #914, #8750 ),
 .UNSPECIFIED., .F., .F. ) 
 B_SPLINE_CURVE_WITH_KNOTS ( ( 3, 2, 2, 2, 2, 2, 2, 2, 2, 2, 2, 2, 2, 2, 2, 2, 2, 2, 2, 2, 2, 2, 2, 2, 2, 2, 2, 2, 2, 2, 2, 2, 2, 2, 2, 2, 2, 2, 2, 2, 2, 2, 2, 2, 2, 2, 2, 2, 2, 2, 2, 2, 2, 2, 2, 2, 2, 2, 2, 2, 3 ),
 ( 0.000000000000000000, 0.01666666666666666644, 0.03333333333333333287, 0.05000000000000000278, 0.06666666666666666574, 0.08333333333333332871, 0.1000000000000000056, 0.1166666666666666685, 0.1333333333333333315, 0.1499999999999999944, 0.1666666666666666574, 0.1833333333333333204, 0.2000000000000000111, 0.2166666666666666741, 0.2333333333333333370, 0.2500000000000000000, 0.2666666666666666630, 0.2833333333333333259, 0.2999999999999999889, 0.3166666666666666519, 0.3333333333333333148, 0.3499999999999999778, 0.3666666666666666408, 0.3833333333333333592, 0.4000000000000000222, 0.4166666666666666852, 0.4333333333333333481, 0.4500000000000000111, 0.4666666666666666741, 0.4833333333333333370, 0.5000000000000000000, 0.5166666666666667185, 0.5333333333333333259, 0.5500000000000000444, 0.5666666666666666519, 0.5833333333333333703, 0.5999999999999999778, 0.6166666666666666963, 0.6333333333333333037, 0.6500000000000000222, 0.6666666666666666297, 0.6833333333333333481, 0.6999999999999999556, 0.7166666666666666741, 0.7333333333333332815, 0.7500000000000000000, 0.7666666666666667185, 0.7833333333333333259, 0.8000000000000000444, 0.8166666666666666519, 0.8333333333333333703, 0.8499999999999999778, 0.8666666666666666963, 0.8833333333333333037, 0.9000000000000000222, 0.9166666666666666297, 0.9333333333333333481, 0.9499999999999999556, 0.9666666666666666741, 0.9833333333333332815, 1.000000000000000000 ),
 .UNSPECIFIED. ) 
 CURVE ( )  GEOMETRIC_REPRESENTATION_ITEM ( )  RATIONAL_B_SPLINE_CURVE ( ( 1.000000000000000000, 0.8660254037844387076, 1.000000000000000000, 0.8660254037844387076, 1.000000000000000000, 0.8660254037844387076, 1.000000000000000000, 0.8660254037844387076, 1.000000000000000000, 0.8660254037844387076, 1.000000000000000000, 0.8660254037844387076, 1.000000000000000000, 0.8660254037844387076, 1.000000000000000000, 0.8660254037844387076, 1.000000000000000000, 0.8660254037844387076, 1.000000000000000000, 0.8660254037844387076, 1.000000000000000000, 0.8660254037844387076, 1.000000000000000000, 0.8660254037844387076, 1.000000000000000000, 0.8660254037844387076, 1.000000000000000000, 0.8660254037844387076, 1.000000000000000000, 0.8660254037844387076, 1.000000000000000000, 0.8660254037844387076, 1.000000000000000000, 0.8660254037844387076, 1.000000000000000000, 0.8660254037844387076, 1.000000000000000000, 0.8660254037844387076, 1.000000000000000000, 0.8660254037844387076, 1.000000000000000000, 0.8660254037844387076, 1.000000000000000000, 0.8660254037844387076, 1.000000000000000000, 0.8660254037844387076, 1.000000000000000000, 0.8660254037844387076, 1.000000000000000000, 0.8660254037844387076, 1.000000000000000000, 0.8660254037844387076, 1.000000000000000000, 0.8660254037844387076, 1.000000000000000000, 0.8660254037844387076, 1.000000000000000000, 0.8660254037844387076, 1.000000000000000000, 0.8660254037844387076, 1.000000000000000000, 0.8660254037844387076, 1.000000000000000000, 0.8660254037844387076, 1.000000000000000000, 0.8660254037844387076, 1.000000000000000000, 0.8660254037844387076, 1.000000000000000000, 0.8660254037844387076, 1.000000000000000000, 0.8660254037844387076, 1.000000000000000000, 0.8660254037844387076, 1.000000000000000000, 0.8660254037844387076, 1.000000000000000000, 0.8660254037844387076, 1.000000000000000000, 0.8660254037844387076, 1.000000000000000000, 0.8660254037844387076, 1.000000000000000000, 0.8660254037844387076, 1.000000000000000000, 0.8660254037844387076, 1.000000000000000000, 0.8660254037844387076, 1.000000000000000000, 0.8660254037844387076, 1.000000000000000000, 0.8660254037844387076, 1.000000000000000000, 0.8660254037844387076, 1.000000000000000000, 0.8660254037844387076, 1.000000000000000000, 0.8660254037844387076, 1.000000000000000000, 0.8660254037844387076, 1.000000000000000000, 0.8660254037844387076, 1.000000000000000000, 0.8660254037844387076, 1.000000000000000000, 0.8660254037844387076, 1.000000000000000000, 0.8660254037844387076, 1.000000000000000000, 0.8660254037844387076, 1.000000000000000000, 0.8660254037844387076, 1.000000000000000000, 0.8660254037844387076, 1.000000000000000000, 0.8660254037844387076, 1.000000000000000000, 0.8660254037844387076, 1.000000000000000000, 0.8660254037844387076, 1.000000000000000000 ) ) 
 REPRESENTATION_ITEM ( '' )  );
#13148=CARTESIAN_POINT ( 'NONE',  ( -1.071796769724485454, 27.11740381056766580, 12.99999999999999467 ) ) ;
#13149=CARTESIAN_POINT ( 'NONE',  ( 3.756430356250002323, 27.46562499938548640, 11.16877607737301226 ) ) ;
#13173=CARTESIAN_POINT ( 'NONE',  ( 3.756430356250004099, 26.97812499938548569, 6.831223922626973533 ) ) ;
#13178=CARTESIAN_POINT ( 'NONE',  ( 3.752267015613588906E-15, 26.40624999877097068, 4.381197846482986158 ) ) ;
#13183=CARTESIAN_POINT ( 'NONE',  ( 1.878215178125004048, 26.22812499938548569, 5.746835883940462963 ) ) ;
#13191=CARTESIAN_POINT ( 'NONE',  ( 4.000000000000003553, 28.99374999877096926, 8.999999999999992895 ) ) ;
#13196=CARTESIAN_POINT ( 'NONE',  ( 3.756430356250003211, 27.87812499938548427, 6.831223922626973533 ) ) ;
#13201=DIRECTION ( 'NONE',  ( -0.000000000000000000, -1.000000000000000000, -0.000000000000000000 ) ) ;
#13209=DIRECTION ( 'NONE',  ( -0.000000000000000000, 1.000000000000000000, -0.000000000000000000 ) ) ;
#13219=CARTESIAN_POINT ( 'NONE',  ( -1.999999999999998224, 29.29374999877096997, 12.46410161513774639 ) ) ;
#13223=DIRECTION ( 'NONE',  ( 1.000000000000000000, 0.000000000000000000, 0.000000000000000000 ) ) ;
#13240=VERTEX_POINT ( 'NONE', #2024 ) ;
#13247=ORIENTED_EDGE ( 'NONE', *, *, #7122, .T. ) ;
#13248=CARTESIAN_POINT ( 'NONE',  ( -1.999999999999998224, 27.55000000000000071, 12.46410161513774639 ) ) ;
#13264=CARTESIAN_POINT ( 'NONE',  ( -3.756430356249995661, 28.14062499938548356, 6.831223922626973533 ) ) ;
#13275=CARTESIAN_POINT ( 'NONE',  ( -3.756430356249995661, 25.32812499938548356, 6.831223922626973533 ) ) ;
#13290=CARTESIAN_POINT ( 'NONE',  ( 3.756430356250002323, 27.35312499938547859, 11.16877607737301226 ) ) ;
#13297=CARTESIAN_POINT ( 'NONE',  ( 4.000000000000003553, 25.43124999877096926, 6.690598923241489970 ) ) ;
#13302=CARTESIAN_POINT ( 'NONE',  ( 3.756430356250002323, 26.11562499938548498, 11.16877607737301403 ) ) ;
#13322=CARTESIAN_POINT ( 'NONE',  ( 4.000000000000003553, 25.88124999877096855, 6.690598923241489970 ) ) ;
#13327=CARTESIAN_POINT ( 'NONE',  ( 3.756430356250003655, 25.25312499938548427, 8.999999999999992895 ) ) ;
#13328=CYLINDRICAL_SURFACE ( 'NONE', #1617, 4.000000000000000000 ) ;
#13334=LINE ( 'NONE', #21310, #18858 ) ;
#13353=CARTESIAN_POINT ( 'NONE',  ( 0.000000000000000000, 0.000000000000000000, 0.000000000000000000 ) ) ;
#13361=CARTESIAN_POINT ( 'NONE',  ( 3.469446951953614189E-15, 40.00000000000000000, 8.999999999999992895 ) ) ;
#13378=CARTESIAN_POINT ( 'NONE',  ( 2.000000000000000888, 26.72500000000000142, 12.46410161513774817 ) ) ;
#13382=CARTESIAN_POINT ( 'NONE',  ( 3.752267015613588906E-15, 27.81250000000000000, 4.381197846482986158 ) ) ;
#13402=CARTESIAN_POINT ( 'NONE',  ( -3.756430356249995661, 28.59062499938548640, 6.831223922626973533 ) ) ;
#13414=FACE_OUTER_BOUND ( 'NONE', #11288, .T. ) ;
#13434=AXIS2_PLACEMENT_3D ( 'NONE', #22586, #16842, #10399 ) ;
#13444=CARTESIAN_POINT ( 'NONE',  ( 3.756430356250002323, 27.01562499938548356, 11.16877607737301403 ) ) ;
#13465=CARTESIAN_POINT ( 'NONE',  ( -3.137519842735244810E-15, 27.30624999877096926, 4.999999999999991118 ) ) ;
#13468=DIRECTION ( 'NONE',  ( 0.000000000000000000, 0.000000000000000000, -1.000000000000000000 ) ) ;
#13471=CARTESIAN_POINT ( 'NONE',  ( -1.878215178124995832, 28.55312499938548498, 5.746835883940462963 ) ) ;
#13504=CARTESIAN_POINT ( 'NONE',  ( -3.999999999999995559, 25.63749999999999929, 6.690598923241487306 ) ) ;
#13518=CARTESIAN_POINT ( 'NONE',  ( 4.000000000000001776, 26.76249999999999929, 11.30940107675849760 ) ) ;
#13536=CARTESIAN_POINT ( 'NONE',  ( -1.878215178124995832, 29.00312499938548427, 5.746835883940462963 ) ) ;
#13539=ORIENTED_EDGE ( 'NONE', *, *, #11589, .T. ) ;
#13557=CARTESIAN_POINT ( 'NONE',  ( -3.137519842735244810E-15, 26.85624999877096641, 4.999999999999991118 ) ) ;
#13559=ADVANCED_FACE ( 'NONE', ( #1718 ), #5371, .T. ) ;
#13589=CARTESIAN_POINT ( 'NONE',  ( 3.756430356250002323, 28.36562499938548854, 11.16877607737301226 ) ) ;
#13594=CARTESIAN_POINT ( 'NONE',  ( 8.831537335106614961E-15, 27.13750000000000284, 12.99999999999999112 ) ) ;
#13616=DIRECTION ( 'NONE',  ( 0.000000000000000000, 0.000000000000000000, -1.000000000000000000 ) ) ;
#13618=CARTESIAN_POINT ( 'NONE',  ( 3.469446951953614189E-15, 40.00000000000000000, 8.999999999999992895 ) ) ;
#13627=ORIENTED_EDGE ( 'NONE', *, *, #24388, .T. ) ;
#13636=CARTESIAN_POINT ( 'NONE',  ( 4.000000000000003553, 27.28749999999999787, 6.690598923241489970 ) ) ;
#13637=CARTESIAN_POINT ( 'NONE',  ( 3.469446951953614189E-15, 40.00000000000000000, 4.999999999999992006 ) ) ;
#13642=DIRECTION ( 'NONE',  ( 0.000000000000000000, 0.000000000000000000, 1.000000000000000000 ) ) ;
#13652=CARTESIAN_POINT ( 'NONE',  ( -3.756430356249997882, 29.56562499938549138, 11.16877607737301226 ) ) ;
#13673=CARTESIAN_POINT ( 'NONE',  ( 3.756430356250002323, 29.15312499938548640, 11.16877607737301226 ) ) ;
#13677=ORIENTED_EDGE ( 'NONE', *, *, #24315, .T. ) ;
#13678=CARTESIAN_POINT ( 'NONE',  ( 4.000000000000001776, 26.25624999877096499, 11.30940107675849760 ) ) ;
#13682=CARTESIAN_POINT ( 'NONE',  ( 3.756430356250003211, 28.44062499938548427, 6.831223922626973533 ) ) ;
#13690=EDGE_CURVE ( 'NONE', #10718, #21413, #3331, .T. ) ;
#13706=CARTESIAN_POINT ( 'NONE',  ( 3.756430356250003655, 28.85312499938548569, 8.999999999999992895 ) ) ;
#13710=ORIENTED_EDGE ( 'NONE', *, *, #12336, .T. ) ;
#13716=ORIENTED_EDGE ( 'NONE', *, *, #9465, .T. ) ;
#13757=CARTESIAN_POINT ( 'NONE',  ( 2.000000000000000888, 26.72500000000000142, 12.46410161513774817 ) ) ;
#13781=CARTESIAN_POINT ( 'NONE',  ( -3.999999999999995559, 26.03124999877097068, 6.690598923241487306 ) ) ;
#13806=CARTESIAN_POINT ( 'NONE',  ( 2.000000000000003997, 28.22500000000000142, 5.535898384862238508 ) ) ;
#13813=CARTESIAN_POINT ( 'NONE',  ( 2.000000000000003997, 26.81874999877096855, 5.535898384862238508 ) ) ;
#13818=CARTESIAN_POINT ( 'NONE',  ( -3.756430356249996105, 29.49062499938548498, 6.831223922626973533 ) ) ;
#13831=CARTESIAN_POINT ( 'NONE',  ( -1.071796769724490117, 27.32634618820330630, 4.999999999999992895 ) ) ;
#13843=CARTESIAN_POINT ( 'NONE',  ( -3.756430356249996994, 27.72812499938548569, 8.999999999999992895 ) ) ;
#13858=EDGE_LOOP ( 'NONE', ( #1742, #11554, #24030, #12957 ) ) ;
#13899=CARTESIAN_POINT ( 'NONE',  ( 3.752267015613588906E-15, 29.16250000000000142, 4.381197846482986158 ) ) ;
#13911=VECTOR ( 'NONE', #7317, 1000.000000000000000 ) ;
#13930=CARTESIAN_POINT ( 'NONE',  ( -3.756430356249997882, 27.65312499938548640, 11.16877607737301226 ) ) ;
#13942=DIRECTION ( 'NONE',  ( -0.000000000000000000, -1.000000000000000000, -0.000000000000000000 ) ) ;
#13947=CARTESIAN_POINT ( 'NONE',  ( 4.000000000000001776, 26.70624999877097139, 11.30940107675849760 ) ) ;
#13952=CARTESIAN_POINT ( 'NONE',  ( 2.672651547586948120E-15, 29.64062499938548356, 13.33755215474603162 ) ) ;
#13976=CARTESIAN_POINT ( 'NONE',  ( 2.672651547586948120E-15, 27.39062499938548356, 13.33755215474602984 ) ) ;
#13995=SHAPE_REPRESENTATION_RELATIONSHIP ( 'NONE' , 'NONE' ,  #20528, #22510 ) ;
#14000=CARTESIAN_POINT ( 'NONE',  ( 8.831537335106614961E-15, 26.63124999877096855, 12.99999999999999112 ) ) ;
#14001=CARTESIAN_POINT ( 'NONE',  ( -1.878215178124995832, 27.09062499938548640, 5.746835883940462963 ) ) ;
#14004=DIRECTION ( 'NONE',  ( -0.000000000000000000, -1.000000000000000000, -0.000000000000000000 ) ) ;
#14015=CARTESIAN_POINT ( 'NONE',  ( 4.143002691484658293E-15, 34.00000000000000000, 14.49999999999999289 ) ) ;
#14017=VERTEX_POINT ( 'NONE', #3512 ) ;
#14023=CARTESIAN_POINT ( 'NONE',  ( 4.000000000000003553, 25.43124999877097281, 6.690598923241489970 ) ) ;
#14036=DIRECTION ( 'NONE',  ( 0.000000000000000000, 1.000000000000000000, 0.000000000000000000 ) ) ;
#14053=CARTESIAN_POINT ( 'NONE',  ( 3.756430356250002323, 27.80312499938548143, 11.16877607737301226 ) ) ;
#14065=DIRECTION ( 'NONE',  ( -0.000000000000000000, -1.000000000000000000, -0.000000000000000000 ) ) ;
#14070=CARTESIAN_POINT ( 'NONE',  ( -3.999999999999997335, 27.00624999877096499, 11.30940107675849404 ) ) ;
#14075=CARTESIAN_POINT ( 'NONE',  ( 1.878215178125000939, 28.77812499938548640, 12.25316411605952283 ) ) ;
#14089=EDGE_CURVE ( 'NONE', #408, #11825, #17633, .T. ) ;
#14098=CARTESIAN_POINT ( 'NONE',  ( -1.878215178124998497, 25.44062499938548427, 12.25316411605951927 ) ) ;
#14103=ORIENTED_EDGE ( 'NONE', *, *, #4123, .T. ) ;
#14119=( BOUNDED_CURVE ( )  B_SPLINE_CURVE ( 2, ( #4839, #11103, #17132, #25103, #20664, #1161, #1300, #13082, #1048 ),
 .UNSPECIFIED., .F., .F. ) 
 B_SPLINE_CURVE_WITH_KNOTS ( ( 3, 2, 2, 2, 3 ),
 ( 0.4750000000000000333, 0.4833333333333333370, 0.5000000000000000000, 0.5166666666666667185, 0.5250000000000000222 ),
 .UNSPECIFIED. ) 
 CURVE ( )  GEOMETRIC_REPRESENTATION_ITEM ( )  RATIONAL_B_SPLINE_CURVE ( ( 0.9330127018922194093, 0.9330127018922196314, 1.000000000000000000, 0.8660254037844387076, 1.000000000000000000, 0.8660254037844387076, 1.000000000000000000, 0.9330127018922194093, 0.9330127018922194093 ) ) 
 REPRESENTATION_ITEM ( '' )  );
#14125=CARTESIAN_POINT ( 'NONE',  ( 3.756430356250003655, 26.94062499938548427, 8.999999999999992895 ) ) ;
#14149=CARTESIAN_POINT ( 'NONE',  ( 4.000000000000001776, 29.01249999999999929, 11.30940107675849760 ) ) ;
#14153=CARTESIAN_POINT ( 'NONE',  ( 3.834746474454188013E-15, 27.75624999877096855, 4.999999999999992006 ) ) ;
#14172=CARTESIAN_POINT ( 'NONE',  ( -3.756430356249996994, 29.52812499938548640, 8.999999999999992895 ) ) ;
#14181=CARTESIAN_POINT ( 'NONE',  ( 3.735045420075836212E-15, 26.15312499938548285, 4.662447845253954171 ) ) ;
#14187=EDGE_CURVE ( 'NONE', #6036, #11726, #23814, .T. ) ;
#14197=CARTESIAN_POINT ( 'NONE',  ( -1.999999999999995781, 25.15000000000000213, 5.535898384862237620 ) ) ;
#14201=CARTESIAN_POINT ( 'NONE',  ( 2.620986760973688460E-15, 28.88124999877096855, 13.61880215351699874 ) ) ;
#14206=CARTESIAN_POINT ( 'NONE',  ( 1.878215178125004048, 28.92812499938548854, 5.746835883940462963 ) ) ;
#14209=CARTESIAN_POINT ( 'NONE',  ( -3.999999999999996447, 27.86874999877096570, 8.999999999999992895 ) ) ;
#14220=CARTESIAN_POINT ( 'NONE',  ( 8.831537335106614961E-15, 27.53124999877097068, 12.99999999999999112 ) ) ;
#14234=CARTESIAN_POINT ( 'NONE',  ( -1.878215178124998497, 25.89062499938548356, 12.25316411605951927 ) ) ;
#14265=CARTESIAN_POINT ( 'NONE',  ( -3.756430356249997438, 25.40312499938548285, 11.16877607737301048 ) ) ;
#14280=ORIENTED_EDGE ( 'NONE', *, *, #24238, .F. ) ;
#14288=( BOUNDED_CURVE ( )  B_SPLINE_CURVE ( 2, ( #24939, #3107, #12520, #1135, #6897, #8871, #18936, #4540, #9108 ),
 .UNSPECIFIED., .F., .F. ) 
 B_SPLINE_CURVE_WITH_KNOTS ( ( 3, 2, 2, 2, 3 ),
 ( 0.8250000000000000666, 0.8333333333333333703, 0.8499999999999999778, 0.8666666666666666963, 0.8750000000000000000 ),
 .UNSPECIFIED. ) 
 CURVE ( )  GEOMETRIC_REPRESENTATION_ITEM ( )  RATIONAL_B_SPLINE_CURVE ( ( 0.9330127018922194093, 0.9330127018922198534, 1.000000000000000000, 0.8660254037844387076, 1.000000000000000000, 0.8660254037844387076, 1.000000000000000000, 0.9330127018922194093, 0.9330127018922194093 ) ) 
 REPRESENTATION_ITEM ( '' )  );
#14310=ORIENTED_EDGE ( 'NONE', *, *, #9465, .F. ) ;
#14323=CARTESIAN_POINT ( 'NONE',  ( 3.756430356250002323, 28.25312499938548427, 11.16877607737301226 ) ) ;
#14333=DIRECTION ( 'NONE',  ( 0.000000000000000000, 1.000000000000000000, 0.000000000000000000 ) ) ;
#14341=CARTESIAN_POINT ( 'NONE',  ( 2.620986760973688460E-15, 27.98124999877096997, 13.61880215351699874 ) ) ;
#14346=CARTESIAN_POINT ( 'NONE',  ( -3.999999999999996447, 28.76874999877096784, 8.999999999999992895 ) ) ;
#14348=CARTESIAN_POINT ( 'NONE',  ( 3.959305671612554781E-15, 40.00000000000000000, 12.99999999999999289 ) ) ;
#14369=CARTESIAN_POINT ( 'NONE',  ( -3.756430356249997882, 26.30312499938548498, 11.16877607737301226 ) ) ;
#14384=ORIENTED_EDGE ( 'NONE', *, *, #16031, .T. ) ;
#14395=CARTESIAN_POINT ( 'NONE',  ( 2.672651547586948120E-15, 26.37812499938548427, 13.33755215474603162 ) ) ;
#14400=CARTESIAN_POINT ( 'NONE',  ( -1.071796769724481901, 28.01740381056766438, 12.99999999999999645 ) ) ;
#14436=CARTESIAN_POINT ( 'NONE',  ( 4.000000000000003553, 25.03750000000000142, 6.690598923241489970 ) ) ;
#14446=CARTESIAN_POINT ( 'NONE',  ( 3.834746474454188013E-15, 28.65624999877096712, 4.999999999999992006 ) ) ;
#14447=CARTESIAN_POINT ( 'NONE',  ( 3.756430356250004099, 26.97812499938548569, 6.831223922626973533 ) ) ;
#14454=CARTESIAN_POINT ( 'NONE',  ( -1.999999999999995781, 26.05000000000000071, 5.535898384862237620 ) ) ;
#14461=CARTESIAN_POINT ( 'NONE',  ( -1.878215178124998497, 26.00312499938548783, 12.25316411605951927 ) ) ;
#14467=CARTESIAN_POINT ( 'NONE',  ( -3.999999999999995559, 25.58124999877096784, 6.690598923241487306 ) ) ;
#14483=CARTESIAN_POINT ( 'NONE',  ( 4.000000000000003553, 27.73750000000000071, 6.690598923241489970 ) ) ;
#14485=CARTESIAN_POINT ( 'NONE',  ( 3.735045420075836212E-15, 26.15312499938548285, 4.662447845253954171 ) ) ;
#14511=CARTESIAN_POINT ( 'NONE',  ( 3.756430356250003655, 25.59062499938548285, 8.999999999999992895 ) ) ;
#14520=VERTEX_POINT ( 'NONE', #9371 ) ;
#14526=VERTEX_POINT ( 'NONE', #17352 ) ;
#14562=CARTESIAN_POINT ( 'NONE',  ( 2.672651547586948120E-15, 29.07812499938548001, 13.33755215474602984 ) ) ;
#14583=CARTESIAN_POINT ( 'NONE',  ( 4.000000000000003553, 29.44374999877096855, 8.999999999999992895 ) ) ;
#14589=FACE_OUTER_BOUND ( 'NONE', #1172, .T. ) ;
#14600=DIRECTION ( 'NONE',  ( -0.000000000000000000, -1.000000000000000000, -0.000000000000000000 ) ) ;
#14613=CARTESIAN_POINT ( 'NONE',  ( 1.878215178125000939, 26.41562499938548214, 12.25316411605952283 ) ) ;
#14633=CARTESIAN_POINT ( 'NONE',  ( -1.071796769724488563, 27.06115380933863435, 12.99999999999999289 ) ) ;
#14644=CARTESIAN_POINT ( 'NONE',  ( 2.672651547586948120E-15, 27.72812499938548569, 13.33755215474603162 ) ) ;
#14651=CARTESIAN_POINT ( 'NONE',  ( -3.999999999999995559, 27.88750000000000284, 6.690598923241487306 ) ) ;
#14660=ORIENTED_EDGE ( 'NONE', *, *, #18061, .F. ) ;
#14666=AXIS2_PLACEMENT_3D ( 'NONE', #21844, #4045, #12289 ) ;
#14673=PRODUCT_DEFINITION_SHAPE ( 'NONE', 'NONE',  #1360 ) ;
#14684=CARTESIAN_POINT ( 'NONE',  ( 1.071796769724487675, 29.14240381056766438, 4.999999999999988454 ) ) ;
#14690=VERTEX_POINT ( 'NONE', #7910 ) ;
#14705=CARTESIAN_POINT ( 'NONE',  ( 3.756430356250002323, 28.70312499938548356, 11.16877607737301226 ) ) ;
#14706=CARTESIAN_POINT ( 'NONE',  ( 4.000000000000003553, 27.23124999877096641, 6.690598923241489970 ) ) ;
#14708=DIRECTION ( 'NONE',  ( -0.000000000000000000, -1.000000000000000000, -0.000000000000000000 ) ) ;
#14714=DIRECTION ( 'NONE',  ( 0.000000000000000000, 0.000000000000000000, 1.000000000000000000 ) ) ;
#14724=CARTESIAN_POINT ( 'NONE',  ( 1.878215178125004048, 25.32812499938548356, 5.746835883940462963 ) ) ;
#14737=DIRECTION ( 'NONE',  ( 0.000000000000000000, 0.000000000000000000, -1.000000000000000000 ) ) ;
#14746=EDGE_CURVE ( 'NONE', #4195, #2907, #13135, .T. ) ;
#14750=CARTESIAN_POINT ( 'NONE',  ( -3.756430356249996994, 27.61562499938548143, 8.999999999999992895 ) ) ;
#14833=CARTESIAN_POINT ( 'NONE',  ( -1.999999999999995781, 26.05000000000000071, 5.535898384862237620 ) ) ;
#14836=CARTESIAN_POINT ( 'NONE',  ( -1.999999999999998224, 26.64999999999999858, 12.46410161513774639 ) ) ;
#14848=CARTESIAN_POINT ( 'NONE',  ( -3.137519842735244810E-15, 26.91249999999999787, 4.999999999999991118 ) ) ;
#14850=CARTESIAN_POINT ( 'NONE',  ( -3.756430356249997882, 25.51562499938548356, 11.16877607737301226 ) ) ;
#14875=CARTESIAN_POINT ( 'NONE',  ( -3.756430356249997882, 28.10312499938548569, 11.16877607737301226 ) ) ;
#14878=DIRECTION ( 'NONE',  ( 0.000000000000000000, 0.000000000000000000, 1.000000000000000000 ) ) ;
#14903=CARTESIAN_POINT ( 'NONE',  ( -1.878215178124995832, 27.99062499938548143, 5.746835883940462963 ) ) ;
#14923=DIRECTION ( 'NONE',  ( -0.000000000000000000, -1.000000000000000000, -0.000000000000000000 ) ) ;
#14953=CARTESIAN_POINT ( 'NONE',  ( 3.756430356250003655, 29.64062499938548356, 8.999999999999992895 ) ) ;
#14956=CARTESIAN_POINT ( 'NONE',  ( -3.999999999999997335, 26.61250000000000071, 11.30940107675849404 ) ) ;
#14960=CARTESIAN_POINT ( 'NONE',  ( -1.999999999999998224, 28.44999999999999929, 12.46410161513774639 ) ) ;
#14971=CARTESIAN_POINT ( 'NONE',  ( 3.756430356250003655, 25.25312499938548427, 8.999999999999992895 ) ) ;
#15000=CARTESIAN_POINT ( 'NONE',  ( 3.756430356250004099, 28.32812499938548356, 6.831223922626973533 ) ) ;
#15012=AXIS2_PLACEMENT_3D ( 'NONE', #20792, #23267, #13088 ) ;
#15031=CARTESIAN_POINT ( 'NONE',  ( 3.756430356250003655, 29.19062499938548072, 8.999999999999992895 ) ) ;
#15037=CARTESIAN_POINT ( 'NONE',  ( 1.878215178125004048, 25.77812499938548640, 5.746835883940462963 ) ) ;
#15090=CARTESIAN_POINT ( 'NONE',  ( -3.999999999999997335, 25.26249999999999929, 11.30940107675849404 ) ) ;
#15111=CARTESIAN_POINT ( 'NONE',  ( -1.999999999999995781, 26.95000000000000284, 5.535898384862237620 ) ) ;
#15112=CARTESIAN_POINT ( 'NONE',  ( 3.756430356250002323, 27.01562499938548356, 11.16877607737301226 ) ) ;
#15116=ORIENTED_EDGE ( 'NONE', *, *, #21632, .T. ) ;
#15143=CARTESIAN_POINT ( 'NONE',  ( 1.878215178125000939, 28.21562499938548640, 12.25316411605952283 ) ) ;
#15149=CARTESIAN_POINT ( 'NONE',  ( -1.999999999999995781, 25.54374999877096997, 5.535898384862237620 ) ) ;
#15154=CARTESIAN_POINT ( 'NONE',  ( 3.834746474454188013E-15, 26.40624999877096357, 4.999999999999992006 ) ) ;
#15169=LINE ( 'NONE', #3376, #11316 ) ;
#15170=CARTESIAN_POINT ( 'NONE',  ( -3.756430356249996105, 28.02812499938548996, 6.831223922626973533 ) ) ;
#15174=CYLINDRICAL_SURFACE ( 'NONE', #24285, 4.000000000000000000 ) ;
#15219=CARTESIAN_POINT ( 'NONE',  ( -3.999999999999996003, 27.43750000000000000, 6.690598923241487306 ) ) ;
#15220=CARTESIAN_POINT ( 'NONE',  ( 4.000000000000003553, 27.19374999877096855, 8.999999999999992895 ) ) ;
#15238=CARTESIAN_POINT ( 'NONE',  ( 2.672651547586948120E-15, 27.84062499938548640, 13.33755215474602984 ) ) ;
#15261=CARTESIAN_POINT ( 'NONE',  ( 3.756430356250002323, 28.25312499938548427, 11.16877607737301226 ) ) ;
#15272=CARTESIAN_POINT ( 'NONE',  ( -1.878215178124995832, 26.75312499938548783, 5.746835883940462963 ) ) ;
#15273=( BOUNDED_CURVE ( )  B_SPLINE_CURVE ( 2, ( #8958, #16932, #24901, #9202, #12862, #17192, #14960, #2931, #11149 ),
 .UNSPECIFIED., .F., .F. ) 
 B_SPLINE_CURVE_WITH_KNOTS ( ( 3, 2, 2, 2, 3 ),
 ( 0.7249999999999999778, 0.7333333333333332815, 0.7500000000000000000, 0.7666666666666667185, 0.7750000000000000222 ),
 .UNSPECIFIED. ) 
 CURVE ( )  GEOMETRIC_REPRESENTATION_ITEM ( )  RATIONAL_B_SPLINE_CURVE ( ( 0.9330127018922194093, 0.9330127018922194093, 1.000000000000000000, 0.8660254037844387076, 1.000000000000000000, 0.8660254037844387076, 1.000000000000000000, 0.9330127018922194093, 0.9330127018922194093 ) ) 
 REPRESENTATION_ITEM ( '' )  );
#15296=CARTESIAN_POINT ( 'NONE',  ( 3.469446951953614189E-15, 46.00000000000000000, 3.499999999999992895 ) ) ;
#15325=CARTESIAN_POINT ( 'NONE',  ( 4.000000000000003553, 25.00000000000000000, 8.999999999999992895 ) ) ;
#15339=CARTESIAN_POINT ( 'NONE',  ( 4.000000000000003553, 28.15000000000000213, 8.999999999999992895 ) ) ;
#15342=FACE_OUTER_BOUND ( 'NONE', #20334, .T. ) ;
#15354=CARTESIAN_POINT ( 'NONE',  ( 1.878215178125000939, 27.87812499938548427, 12.25316411605952283 ) ) ;
#15367=( BOUNDED_CURVE ( )  B_SPLINE_CURVE ( 2, ( #10302, #18294, #8617, #2463, #24173, #262, #4429, #14633, #8494 ),
 .UNSPECIFIED., .F., .F. ) 
 B_SPLINE_CURVE_WITH_KNOTS ( ( 3, 2, 2, 2, 3 ),
 ( 0.3250000000000000111, 0.3333333333333333148, 0.3499999999999999778, 0.3666666666666666408, 0.3750000000000000000 ),
 .UNSPECIFIED. ) 
 CURVE ( )  GEOMETRIC_REPRESENTATION_ITEM ( )  RATIONAL_B_SPLINE_CURVE ( ( 0.9330127018922194093, 0.9330127018922196314, 1.000000000000000000, 0.8660254037844387076, 1.000000000000000000, 0.8660254037844387076, 1.000000000000000000, 0.9330127018922194093, 0.9330127018922194093 ) ) 
 REPRESENTATION_ITEM ( '' )  );
#15385=CARTESIAN_POINT ( 'NONE',  ( 2.620986760973688460E-15, 26.18124999877096926, 13.61880215351699874 ) ) ;
#15389=PLANE ( 'NONE',  #10412 ) ;
#15391=CARTESIAN_POINT ( 'NONE',  ( -1.878215178124998497, 26.45312499938548711, 12.25316411605951927 ) ) ;
#15404=CARTESIAN_POINT ( 'NONE',  ( 4.000000000000003553, 29.03124999877096712, 6.690598923241489970 ) ) ;
#15413=CARTESIAN_POINT ( 'NONE',  ( 4.000000000000001776, 25.80624999877096926, 11.30940107675849760 ) ) ;
#15452=DIRECTION ( 'NONE',  ( -0.000000000000000000, -1.000000000000000000, -0.000000000000000000 ) ) ;
#15473=CARTESIAN_POINT ( 'NONE',  ( -3.999999999999996447, 28.37500000000000000, 8.999999999999992895 ) ) ;
#15481=DIRECTION ( 'NONE',  ( 0.000000000000000000, 0.000000000000000000, -1.000000000000000000 ) ) ;
#15485=STYLED_ITEM('',(#25928),#22659);
#15496=CARTESIAN_POINT ( 'NONE',  ( 2.672651547586948120E-15, 28.29062499938548569, 13.33755215474602984 ) ) ;
#15506=CARTESIAN_POINT ( 'NONE',  ( -3.756430356249997882, 25.85312499938548925, 11.16877607737301226 ) ) ;
#15523=CARTESIAN_POINT ( 'NONE',  ( 3.735045420075836212E-15, 29.30312499938548498, 4.662447845253954171 ) ) ;
#15529=CARTESIAN_POINT ( 'NONE',  ( 4.000000000000003553, 26.78124999877097068, 6.690598923241489970 ) ) ;
#15531=FACE_BOUND ( 'NONE', #8215, .T. ) ;
#15533=CARTESIAN_POINT ( 'NONE',  ( 3.735045420075836212E-15, 27.16562499938547859, 4.662447845253954171 ) ) ;
#15556=CARTESIAN_POINT ( 'NONE',  ( -3.756430356249996994, 27.27812499938548640, 8.999999999999992895 ) ) ;
#15558=FACE_OUTER_BOUND ( 'NONE', #4294, .T. ) ;
#15561=DIRECTION ( 'NONE',  ( -0.000000000000000000, -1.000000000000000000, -0.000000000000000000 ) ) ;
#15565=ORIENTED_EDGE ( 'NONE', *, *, #14187, .F. ) ;
#15595=ORIENTED_EDGE ( 'NONE', *, *, #21632, .F. ) ;
#15605=( GEOMETRIC_REPRESENTATION_CONTEXT ( 3 ) GLOBAL_UNCERTAINTY_ASSIGNED_CONTEXT ( ( #6796 ) ) GLOBAL_UNIT_ASSIGNED_CONTEXT ( ( #9926, #16483, #5884 ) ) REPRESENTATION_CONTEXT ( 'NONE', 'WORKASPACE' ) );
#15607=CARTESIAN_POINT ( 'NONE',  ( 4.000000000000003553, 26.35000000000000142, 8.999999999999992895 ) ) ;
#15616=CARTESIAN_POINT ( 'NONE',  ( -1.999999999999998224, 29.35000000000000142, 12.46410161513774639 ) ) ;
#15627=CARTESIAN_POINT ( 'NONE',  ( 3.756430356250002323, 27.91562499938548569, 11.16877607737301226 ) ) ;
#15648=( BOUNDED_CURVE ( )  B_SPLINE_CURVE ( 2, ( #473, #6207, #14197, #16430, #5961, #7916, #8058, #6344, #24121 ),
 .UNSPECIFIED., .F., .F. ) 
 B_SPLINE_CURVE_WITH_KNOTS ( ( 3, 2, 2, 2, 3 ),
 ( 0.02500000000000000139, 0.03333333333333333287, 0.05000000000000000278, 0.06666666666666666574, 0.07500000000000001110 ),
 .UNSPECIFIED. ) 
 CURVE ( )  GEOMETRIC_REPRESENTATION_ITEM ( )  RATIONAL_B_SPLINE_CURVE ( ( 0.9330127018922194093, 0.9330127018922194093, 1.000000000000000000, 0.8660254037844387076, 1.000000000000000000, 0.8660254037844387076, 1.000000000000000000, 0.9330127018922191873, 0.9330127018922192983 ) ) 
 REPRESENTATION_ITEM ( '' )  );
#15655=CARTESIAN_POINT ( 'NONE',  ( 4.000000000000003553, 26.74374999877096926, 8.999999999999992895 ) ) ;
#15659=CARTESIAN_POINT ( 'NONE',  ( -3.756430356249997438, 27.76562499938549067, 11.16877607737301048 ) ) ;
#15680=CARTESIAN_POINT ( 'NONE',  ( 3.756430356250003655, 28.40312499938548640, 8.999999999999992895 ) ) ;
#15684=ORIENTED_EDGE ( 'NONE', *, *, #11818, .T. ) ;
#15703=DIRECTION ( 'NONE',  ( 0.000000000000000000, 0.000000000000000000, 1.000000000000000000 ) ) ;
#15723=ORIENTED_EDGE ( 'NONE', *, *, #10240, .T. ) ;
#15728=CARTESIAN_POINT ( 'NONE',  ( -3.999999999999996003, 27.88750000000000284, 6.690598923241487306 ) ) ;
#15733=LINE ( 'NONE', #23189, #9993 ) ;
#15735=CARTESIAN_POINT ( 'NONE',  ( 3.469446951953614189E-15, 46.00000000000000000, 8.999999999999992895 ) ) ;
#15754=CARTESIAN_POINT ( 'NONE',  ( 2.672651547586948120E-15, 25.47812499938548569, 13.33755215474602984 ) ) ;
#15767=CARTESIAN_POINT ( 'NONE',  ( 1.878215178125000939, 29.11562499938548498, 12.25316411605952283 ) ) ;
#15771=CARTESIAN_POINT ( 'NONE',  ( 4.000000000000003553, 28.54374999877096997, 8.999999999999992895 ) ) ;
#15773=DIRECTION ( 'NONE',  ( 0.000000000000000000, 1.000000000000000000, 0.000000000000000000 ) ) ;
#15775=CARTESIAN_POINT ( 'NONE',  ( 1.878215178125004048, 29.37812499938548783, 5.746835883940462963 ) ) ;
#15800=CARTESIAN_POINT ( 'NONE',  ( 1.878215178125000939, 27.87812499938548427, 12.25316411605952283 ) ) ;
#15816=VERTEX_POINT ( 'NONE', #1857 ) ;
#15826=CARTESIAN_POINT ( 'NONE',  ( 3.878215178125003604, 29.57031249969274356, 8.999999999999992895 ) ) ;
#15860=CARTESIAN_POINT ( 'NONE',  ( 3.469446951953614189E-15, 40.00000000000000000, 8.999999999999992895 ) ) ;
#15877=CARTESIAN_POINT ( 'NONE',  ( 1.878215178125000939, 29.22812499938548569, 12.25316411605952283 ) ) ;
#15878=CARTESIAN_POINT ( 'NONE',  ( 2.000000000000000888, 28.01874999877096784, 12.46410161513774817 ) ) ;
#15901=CARTESIAN_POINT ( 'NONE',  ( 1.071796769724487675, 29.53615380933863221, 4.999999999999988454 ) ) ;
#15907=CARTESIAN_POINT ( 'NONE',  ( -1.999999999999998224, 27.04374999877096641, 12.46410161513774639 ) ) ;
#15912=CARTESIAN_POINT ( 'NONE',  ( 3.756430356250003211, 27.54062499938547859, 6.831223922626973533 ) ) ;
#15917=ORIENTED_EDGE ( 'NONE', *, *, #11622, .T. ) ;
#15939=CARTESIAN_POINT ( 'NONE',  ( -1.878215178124995832, 26.75312499938548783, 5.746835883940462963 ) ) ;
#15972=CARTESIAN_POINT ( 'NONE',  ( -1.878215178124998497, 25.89062499938548356, 12.25316411605951927 ) ) ;
#16004=EDGE_CURVE ( 'NONE', #22149, #10879, #12975, .T. ) ;
#16005=CARTESIAN_POINT ( 'NONE',  ( -1.057460391440397258E-14, 29.16249999999999787, 4.999999999999992006 ) ) ;
#16013=CARTESIAN_POINT ( 'NONE',  ( -1.071796769724488563, 26.16115380933863221, 12.99999999999999289 ) ) ;
#16023=CARTESIAN_POINT ( 'NONE',  ( 3.756430356250003655, 26.49062499938548498, 8.999999999999992895 ) ) ;
#16027=CARTESIAN_POINT ( 'NONE',  ( 3.469446951953614189E-15, 46.00000000000000000, 3.499999999999992895 ) ) ;
#16031=EDGE_CURVE ( 'NONE', #22942, #21859, #14119, .T. ) ;
#16039=LINE ( 'NONE', #24000, #1745 ) ;
#16044=CARTESIAN_POINT ( 'NONE',  ( 2.620986760973688460E-15, 27.53124999877097068, 13.61880215351699874 ) ) ;
#16048=CARTESIAN_POINT ( 'NONE',  ( -3.756430356249997438, 28.21562499938548640, 11.16877607737301048 ) ) ;
#16061=PRODUCT_DEFINITION_FORMATION_WITH_SPECIFIED_SOURCE ( 'ANY', '', #22379, .NOT_KNOWN. ) ;
#16070=CARTESIAN_POINT ( 'NONE',  ( 1.878215178125000939, 29.67812499938548498, 12.25316411605952283 ) ) ;
#16079=DIRECTION ( 'NONE',  ( 0.000000000000000000, 0.000000000000000000, -1.000000000000000000 ) ) ;
#16091=CARTESIAN_POINT ( 'NONE',  ( 3.469446951953614189E-15, 34.00000000000000000, 8.999999999999992895 ) ) ;
#16094=CARTESIAN_POINT ( 'NONE',  ( 1.878215178125000939, 27.31562499938548427, 12.25316411605952283 ) ) ;
#16109=VERTEX_POINT ( 'NONE', #7051 ) ;
#16117=CARTESIAN_POINT ( 'NONE',  ( 2.000000000000003997, 29.12500000000000000, 5.535898384862238508 ) ) ;
#16129=CARTESIAN_POINT ( 'NONE',  ( 4.000000000000003553, 29.08750000000000213, 6.690598923241489970 ) ) ;
#16136=ADVANCED_FACE ( 'NONE', ( #22881 ), #5104, .F. ) ;
#16140=CARTESIAN_POINT ( 'NONE',  ( 2.672651547586948120E-15, 29.64062499938548356, 13.33755215474602984 ) ) ;
#16147=CARTESIAN_POINT ( 'NONE',  ( -1.878215178124995832, 27.99062499938548143, 5.746835883940462963 ) ) ;
#16150=CARTESIAN_POINT ( 'NONE',  ( 1.859271017917182139E-15, 28.88124999877096499, 12.99999999999999289 ) ) ;
#16162=CARTESIAN_POINT ( 'NONE',  ( -3.999999999999996447, 28.76874999877096784, 8.999999999999992895 ) ) ;
#16166=CARTESIAN_POINT ( 'NONE',  ( 3.756430356250003211, 28.89062499938548356, 6.831223922626973533 ) ) ;
#16168=CARTESIAN_POINT ( 'NONE',  ( -1.071796769724481901, 27.96115380933863293, 12.99999999999999645 ) ) ;
#16177=CARTESIAN_POINT ( 'NONE',  ( 1.859271017917182139E-15, 25.78750000000000142, 12.99999999999999289 ) ) ;
#16182=EDGE_CURVE ( 'NONE', #16109, #19025, #9456, .T. ) ;
#16187=CARTESIAN_POINT ( 'NONE',  ( 3.756430356250002323, 29.71562499938548640, 11.16877607737301226 ) ) ;
#16189=VERTEX_POINT ( 'NONE', #9523 ) ;
#16199=ORIENTED_EDGE ( 'NONE', *, *, #20025, .F. ) ;
#16204=CARTESIAN_POINT ( 'NONE',  ( -1.071796769724485454, 26.61115380933863150, 12.99999999999999467 ) ) ;
#16205=ADVANCED_FACE ( 'NONE', ( #15558 ), #13328, .T. ) ;
#16215=CARTESIAN_POINT ( 'NONE',  ( 3.756430356250002323, 26.90312499938548285, 11.16877607737301403 ) ) ;
#16260=( BOUNDED_CURVE ( )  B_SPLINE_CURVE ( 2, ( #10222, #9617, #5689, #22002, #4079, #16129, #6173, #14684, #12974 ),
 .UNSPECIFIED., .F., .F. ) 
 B_SPLINE_CURVE_WITH_KNOTS ( ( 3, 2, 2, 2, 3 ),
 ( 0.8750000000000000000, 0.8833333333333333037, 0.9000000000000000222, 0.9166666666666666297, 0.9250000000000000444 ),
 .UNSPECIFIED. ) 
 CURVE ( )  GEOMETRIC_REPRESENTATION_ITEM ( )  RATIONAL_B_SPLINE_CURVE ( ( 0.9330127018922194093, 0.9330127018922194093, 1.000000000000000000, 0.8660254037844387076, 1.000000000000000000, 0.8660254037844387076, 1.000000000000000000, 0.9330127018922189652, 0.9330127018922194093 ) ) 
 REPRESENTATION_ITEM ( '' )  );
#16271=CARTESIAN_POINT ( 'NONE',  ( 2.000000000000000888, 28.46874999877097068, 12.46410161513774817 ) ) ;
#16273=CARTESIAN_POINT ( 'NONE',  ( 3.756430356250004099, 26.52812499938548285, 6.831223922626973533 ) ) ;
#16294=CARTESIAN_POINT ( 'NONE',  ( 4.000000000000003553, 28.13124999877096855, 6.690598923241489970 ) ) ;
#16325=CARTESIAN_POINT ( 'NONE',  ( -3.756430356249996994, 29.52812499938548640, 8.999999999999992895 ) ) ;
#16357=CARTESIAN_POINT ( 'NONE',  ( 3.756430356250002323, 27.35312499938547859, 11.16877607737301403 ) ) ;
#16366=CARTESIAN_POINT ( 'NONE',  ( -1.999999999999995781, 27.85000000000000142, 5.535898384862237620 ) ) ;
#16375=EDGE_LOOP ( 'NONE', ( #19175, #20041, #9950, #4758 ) ) ;
#16379=ORIENTED_EDGE ( 'NONE', *, *, #20965, .T. ) ;
#16415=CARTESIAN_POINT ( 'NONE',  ( -1.878215178124995832, 27.09062499938548640, 5.746835883940462963 ) ) ;
#16430=CARTESIAN_POINT ( 'NONE',  ( -3.999999999999995559, 25.18750000000000000, 6.690598923241487306 ) ) ;
#16435=CARTESIAN_POINT ( 'NONE',  ( -3.756430356249996994, 25.92812499938548498, 8.999999999999992895 ) ) ;
#16442=CARTESIAN_POINT ( 'NONE',  ( 3.834746474454188013E-15, 27.75624999877096855, 4.999999999999992006 ) ) ;
#16461=CARTESIAN_POINT ( 'NONE',  ( -3.756430356249995661, 25.32812499938548356, 6.831223922626973533 ) ) ;
#16477=ORIENTED_EDGE ( 'NONE', *, *, #14746, .T. ) ;
#16483=( NAMED_UNIT ( * ) PLANE_ANGLE_UNIT ( ) SI_UNIT ( $, .RADIAN. ) );
#16488=CARTESIAN_POINT ( 'NONE',  ( 3.735045420075836212E-15, 25.70312499938548001, 4.662447845253954171 ) ) ;
#16535=LINE ( 'NONE', #21323, #6918 ) ;
#16539=CARTESIAN_POINT ( 'NONE',  ( 3.756430356250002323, 26.90312499938548640, 11.16877607737301226 ) ) ;
#16555=CARTESIAN_POINT ( 'NONE',  ( -1.999999999999998224, 29.74374999877096926, 12.46410161513774639 ) ) ;
#16579=CARTESIAN_POINT ( 'NONE',  ( 3.756430356250002323, 25.55312499938548143, 11.16877607737301226 ) ) ;
#16591=ORIENTED_EDGE ( 'NONE', *, *, #11468, .T. ) ;
#16604=CARTESIAN_POINT ( 'NONE',  ( 3.756430356250002323, 29.15312499938548640, 11.16877607737301403 ) ) ;
#16623=CARTESIAN_POINT ( 'NONE',  ( 3.959305671612554781E-15, 40.00000000000000000, 12.99999999999999289 ) ) ;
#16627=APPLICATION_CONTEXT ( 'automotive_design' ) ;
#16651=ORIENTED_EDGE ( 'NONE', *, *, #2772, .T. ) ;
#16657=CARTESIAN_POINT ( 'NONE',  ( -3.756430356249997882, 29.00312499938548072, 11.16877607737301226 ) ) ;
#16658=CARTESIAN_POINT ( 'NONE',  ( 2.000000000000000888, 27.11874999877096926, 12.46410161513774817 ) ) ;
#16677=CARTESIAN_POINT ( 'NONE',  ( 1.878215178125000939, 26.07812499938548356, 12.25316411605952283 ) ) ;
#16681=ORIENTED_EDGE ( 'NONE', *, *, #14746, .F. ) ;
#16691=FACE_OUTER_BOUND ( 'NONE', #632, .T. ) ;
#16695=CARTESIAN_POINT ( 'NONE',  ( 3.469446951953614189E-15, 40.00000000000000000, 8.999999999999992895 ) ) ;
#16705=CARTESIAN_POINT ( 'NONE',  ( 1.878215178125000939, 28.66562499938548569, 12.25316411605952283 ) ) ;
#16740=CARTESIAN_POINT ( 'NONE',  ( 1.878215178125004048, 27.91562499938548569, 5.746835883940462963 ) ) ;
#16802=CARTESIAN_POINT ( 'NONE',  ( -3.999999999999996447, 25.67500000000000071, 8.999999999999992895 ) ) ;
#16817=AXIS2_PLACEMENT_3D ( 'NONE', #18360, #11947, #24502 ) ;
#16820=CARTESIAN_POINT ( 'NONE',  ( -3.756430356249995661, 26.34062499938548285, 6.831223922626973533 ) ) ;
#16822=VERTEX_POINT ( 'NONE', #18248 ) ;
#16833=EDGE_CURVE ( 'NONE', #24266, #6036, #15648, .T. ) ;
#16842=DIRECTION ( 'NONE',  ( -0.000000000000000000, -1.000000000000000000, -0.000000000000000000 ) ) ;
#16850=CARTESIAN_POINT ( 'NONE',  ( 1.878215178125004048, 27.91562499938548569, 5.746835883940462963 ) ) ;
#16878=CARTESIAN_POINT ( 'NONE',  ( 1.878215178125000939, 28.21562499938548640, 12.25316411605952283 ) ) ;
#16884=CARTESIAN_POINT ( 'NONE',  ( 3.756430356250003655, 26.15312499938548640, 8.999999999999992895 ) ) ;
#16906=CARTESIAN_POINT ( 'NONE',  ( 3.469446951953614189E-15, 34.00000000000000000, 4.999999999999992006 ) ) ;
#16918=ORIENTED_EDGE ( 'NONE', *, *, #3594, .T. ) ;
#16927=CARTESIAN_POINT ( 'NONE',  ( -3.756430356249997882, 28.55312499938548498, 11.16877607737301226 ) ) ;
#16932=CARTESIAN_POINT ( 'NONE',  ( -1.071796769724487230, 28.28259618943233988, 4.999999999999992006 ) ) ;
#16937=VERTEX_POINT ( 'NONE', #14015 ) ;
#16941=CARTESIAN_POINT ( 'NONE',  ( -3.999999999999997335, 27.06250000000000000, 11.30940107675849404 ) ) ;
#16942=CARTESIAN_POINT ( 'NONE',  ( 2.000000000000000888, 29.36874999877096926, 12.46410161513774817 ) ) ;
#16949=CARTESIAN_POINT ( 'NONE',  ( 1.071796769724494558, 26.38615380933864074, 4.999999999999992895 ) ) ;
#16967=CARTESIAN_POINT ( 'NONE',  ( -3.756430356249997882, 27.65312499938548640, 11.16877607737301226 ) ) ;
#16979=CARTESIAN_POINT ( 'NONE',  ( 3.735045420075836212E-15, 26.71562499938548285, 4.662447845253954171 ) ) ;
#16988=CARTESIAN_POINT ( 'NONE',  ( 2.000000000000000888, 28.91874999877096997, 12.46410161513774817 ) ) ;
#16996=CARTESIAN_POINT ( 'NONE',  ( -1.878215178124995832, 27.54062499938548214, 5.746835883940462963 ) ) ;
#16999=DIRECTION ( 'NONE',  ( 0.000000000000000000, 1.000000000000000000, 0.000000000000000000 ) ) ;
#17002=CARTESIAN_POINT ( 'NONE',  ( 2.672651547586948120E-15, 25.59062499938548640, 13.33755215474602984 ) ) ;
#17045=CARTESIAN_POINT ( 'NONE',  ( -3.999999999999996447, 25.22500000000000142, 8.999999999999992895 ) ) ;
#17053=( BOUNDED_CURVE ( )  B_SPLINE_CURVE ( 2, ( #23876, #21786, #5821, #25321, #17858, #11456, #13806, #5577, #7527 ),
 .UNSPECIFIED., .F., .F. ) 
 B_SPLINE_CURVE_WITH_KNOTS ( ( 3, 2, 2, 2, 3 ),
 ( 0.6750000000000000444, 0.6833333333333333481, 0.6999999999999999556, 0.7166666666666666741, 0.7249999999999999778 ),
 .UNSPECIFIED. ) 
 CURVE ( )  GEOMETRIC_REPRESENTATION_ITEM ( )  RATIONAL_B_SPLINE_CURVE ( ( 0.9330127018922194093, 0.9330127018922198534, 1.000000000000000000, 0.8660254037844387076, 1.000000000000000000, 0.8660254037844387076, 1.000000000000000000, 0.9330127018922194093, 0.9330127018922194093 ) ) 
 REPRESENTATION_ITEM ( '' )  );
#17063=CARTESIAN_POINT ( 'NONE',  ( -3.756430356249997882, 27.31562499938548427, 11.16877607737301226 ) ) ;
#17071=CARTESIAN_POINT ( 'NONE',  ( 2.000000000000000888, 26.21874999877096712, 12.46410161513774817 ) ) ;
#17085=DIRECTION ( 'NONE',  ( 0.000000000000000000, 0.000000000000000000, -1.000000000000000000 ) ) ;
#17092=CARTESIAN_POINT ( 'NONE',  ( 3.756430356250004099, 27.42812499938548143, 6.831223922626973533 ) ) ;
#17097=CARTESIAN_POINT ( 'NONE',  ( -3.999999999999997335, 25.65624999877097068, 11.30940107675849404 ) ) ;
#17102=CARTESIAN_POINT ( 'NONE',  ( 2.672651547586948120E-15, 26.49062499938548498, 13.33755215474603162 ) ) ;
#17124=CARTESIAN_POINT ( 'NONE',  ( 3.756430356250003211, 28.77812499938548285, 6.831223922626973533 ) ) ;
#17127=CARTESIAN_POINT ( 'NONE',  ( 3.959305671612554781E-15, 40.00000000000000000, 12.99999999999999289 ) ) ;
#17132=CARTESIAN_POINT ( 'NONE',  ( 2.000000000000000888, 27.56874999877096855, 12.46410161513774817 ) ) ;
#17141=ORIENTED_EDGE ( 'NONE', *, *, #3927, .T. ) ;
#17144=ORIENTED_EDGE ( 'NONE', *, *, #20699, .F. ) ;
#17183=CARTESIAN_POINT ( 'NONE',  ( 3.752267015613588906E-15, 27.36250000000000071, 4.381197846482986158 ) ) ;
#17192=CARTESIAN_POINT ( 'NONE',  ( -3.999999999999997335, 28.41250000000000142, 11.30940107675849404 ) ) ;
#17206=CARTESIAN_POINT ( 'NONE',  ( -3.756430356249996994, 26.82812499938548711, 8.999999999999992895 ) ) ;
#17207=VECTOR ( 'NONE', #10209, 1000.000000000000000 ) ;
#17222=ADVANCED_FACE ( 'NONE', ( #24855 ), #19211, .T. ) ;
#17224=SHAPE_DEFINITION_REPRESENTATION ( #14673, #20528 ) ;
#17234=CARTESIAN_POINT ( 'NONE',  ( 3.756430356250003655, 28.29062499938548569, 8.999999999999992895 ) ) ;
#17240=FACE_OUTER_BOUND ( 'NONE', #25733, .T. ) ;
#17245=CARTESIAN_POINT ( 'NONE',  ( -3.756430356249997438, 26.41562499938548569, 11.16877607737301048 ) ) ;
#17271=DIRECTION ( 'NONE',  ( -1.000000000000000000, 0.000000000000000000, -0.000000000000000000 ) ) ;
#17317=CARTESIAN_POINT ( 'NONE',  ( 2.620986760973688460E-15, 28.03750000000000142, 13.61880215351699874 ) ) ;
#17318=FACE_OUTER_BOUND ( 'NONE', #16375, .T. ) ;
#17333=CARTESIAN_POINT ( 'NONE',  ( -3.756430356249997882, 28.66562499938548569, 11.16877607737301226 ) ) ;
#17352=CARTESIAN_POINT ( 'NONE',  ( -1.057460391440397258E-14, 29.16249999999999787, 4.999999999999992006 ) ) ;
#17361=CARTESIAN_POINT ( 'NONE',  ( 4.000000000000001776, 25.80624999877096926, 11.30940107675849760 ) ) ;
#17365=ORIENTED_EDGE ( 'NONE', *, *, #7727, .T. ) ;
#17366=CARTESIAN_POINT ( 'NONE',  ( 2.672651547586948120E-15, 26.04062499938548925, 13.33755215474603162 ) ) ;
#17391=CARTESIAN_POINT ( 'NONE',  ( 1.071796769724494558, 27.34240381056766722, 4.999999999999992895 ) ) ;
#17394=ORIENTED_EDGE ( 'NONE', *, *, #20992, .F. ) ;
#17426=ORIENTED_EDGE ( 'NONE', *, *, #23054, .F. ) ;
#17431=CARTESIAN_POINT ( 'NONE',  ( 2.000000000000003997, 27.32500000000000284, 5.535898384862238508 ) ) ;
#17445=ORIENTED_EDGE ( 'NONE', *, *, #25119, .T. ) ;
#17447=CARTESIAN_POINT ( 'NONE',  ( 3.756430356250003655, 28.85312499938548569, 8.999999999999992895 ) ) ;
#17455=CARTESIAN_POINT ( 'NONE',  ( -1.878215178124995832, 25.74062499938548498, 5.746835883940462963 ) ) ;
#17481=CARTESIAN_POINT ( 'NONE',  ( -1.878215178124995832, 25.85312499938548569, 5.746835883940462963 ) ) ;
#17497=CARTESIAN_POINT ( 'NONE',  ( 2.000000000000003997, 25.91874999877096997, 5.535898384862238508 ) ) ;
#17502=CARTESIAN_POINT ( 'NONE',  ( 3.469446951953614189E-15, 40.00000000000000000, 8.999999999999992895 ) ) ;
#17504=CARTESIAN_POINT ( 'NONE',  ( 3.756430356250003655, 26.60312499938548569, 8.999999999999992895 ) ) ;
#17544=ADVANCED_FACE ( 'NONE', ( #8485 ), #20113, .T. ) ;
#17546=AXIS2_PLACEMENT_3D ( 'NONE', #10043, #1949, #8099 ) ;
#17558=CARTESIAN_POINT ( 'NONE',  ( 1.071796769724491227, 26.89240381056766793, 4.999999999999989342 ) ) ;
#17561=CARTESIAN_POINT ( 'NONE',  ( -3.999999999999997335, 26.16250000000000142, 11.30940107675849404 ) ) ;
#17568=CYLINDRICAL_SURFACE ( 'NONE', #21338, 4.000000000000000000 ) ;
#17572=CARTESIAN_POINT ( 'NONE',  ( 1.859271017917182139E-15, 25.78750000000000142, 12.99999999999999289 ) ) ;
#17579=CARTESIAN_POINT ( 'NONE',  ( 1.859271017917182139E-15, 29.78124999877096712, 12.99999999999999289 ) ) ;
#17581=CARTESIAN_POINT ( 'NONE',  ( 3.756430356250002323, 28.36562499938548854, 11.16877607737301226 ) ) ;
#17590=CARTESIAN_POINT ( 'NONE',  ( 2.672651547586948120E-15, 25.92812499938548498, 13.33755215474602984 ) ) ;
#17602=DIRECTION ( 'NONE',  ( 0.000000000000000000, 0.000000000000000000, -1.000000000000000000 ) ) ;
#17609=CARTESIAN_POINT ( 'NONE',  ( -3.137519842735244810E-15, 26.85624999877096641, 4.999999999999991118 ) ) ;
#17613=CARTESIAN_POINT ( 'NONE',  ( -1.878215178124998497, 27.80312499938548498, 12.25316411605951927 ) ) ;
#17628=( BOUNDED_CURVE ( )  B_SPLINE_CURVE ( 2, ( #17572, #8021, #25547, #7633, #8151, #19512, #8410, #4472, #24367 ),
 .UNSPECIFIED., .F., .F. ) 
 B_SPLINE_CURVE_WITH_KNOTS ( ( 3, 2, 2, 2, 3 ),
 ( 0.1749999999999999889, 0.1833333333333333204, 0.2000000000000000111, 0.2166666666666666741, 0.2250000000000000056 ),
 .UNSPECIFIED. ) 
 CURVE ( )  GEOMETRIC_REPRESENTATION_ITEM ( )  RATIONAL_B_SPLINE_CURVE ( ( 0.9330127018922194093, 0.9330127018922194093, 1.000000000000000000, 0.8660254037844387076, 1.000000000000000000, 0.8660254037844387076, 1.000000000000000000, 0.9330127018922194093, 0.9330127018922194093 ) ) 
 REPRESENTATION_ITEM ( '' )  );
#17633=( BOUNDED_CURVE ( )  B_SPLINE_CURVE ( 2, ( #9781, #3378, #3761, #15413, #19576, #13322, #17497, #25476, #23386 ),
 .UNSPECIFIED., .F., .F. ) 
 B_SPLINE_CURVE_WITH_KNOTS ( ( 3, 2, 2, 2, 3 ),
 ( 0.07500000000000001110, 0.08333333333333332871, 0.1000000000000000056, 0.1166666666666666685, 0.1250000000000000000 ),
 .UNSPECIFIED. ) 
 CURVE ( )  GEOMETRIC_REPRESENTATION_ITEM ( )  RATIONAL_B_SPLINE_CURVE ( ( 0.9330127018922192983, 0.9330127018922194093, 1.000000000000000000, 0.8660254037844387076, 1.000000000000000000, 0.8660254037844387076, 1.000000000000000000, 0.9330127018922194093, 0.9330127018922194093 ) ) 
 REPRESENTATION_ITEM ( '' )  );
#17645=CARTESIAN_POINT ( 'NONE',  ( 1.878215178125000939, 26.52812499938548285, 12.25316411605952283 ) ) ;
#17652=PLANE ( 'NONE',  #11341 ) ;
#17653=FACE_OUTER_BOUND ( 'NONE', #21802, .T. ) ;
#17697=CARTESIAN_POINT ( 'NONE',  ( -1.999999999999998224, 26.64999999999999858, 12.46410161513774639 ) ) ;
#17704=DIRECTION ( 'NONE',  ( -0.000000000000000000, -1.000000000000000000, -0.000000000000000000 ) ) ;
#17724=FACE_OUTER_BOUND ( 'NONE', #20199, .T. ) ;
#17730=CARTESIAN_POINT ( 'NONE',  ( -3.999999999999995559, 27.43750000000000000, 6.690598923241487306 ) ) ;
#17735=CARTESIAN_POINT ( 'NONE',  ( 2.672651547586948120E-15, 29.52812499938548285, 13.33755215474602984 ) ) ;
#17739=ORIENTED_EDGE ( 'NONE', *, *, #20348, .F. ) ;
#17740=CARTESIAN_POINT ( 'NONE',  ( 2.620986760973688460E-15, 28.43124999877096926, 13.61880215351699874 ) ) ;
#17744=CARTESIAN_POINT ( 'NONE',  ( 3.756430356250003211, 29.34062499938548640, 6.831223922626973533 ) ) ;
#17753=CARTESIAN_POINT ( 'NONE',  ( -1.999999999999995781, 27.34374999877097068, 5.535898384862237620 ) ) ;
#17767=CARTESIAN_POINT ( 'NONE',  ( 1.878215178125000939, 28.32812499938548711, 12.25316411605952283 ) ) ;
#17785=CARTESIAN_POINT ( 'NONE',  ( -1.071796769724487230, 26.42634618820330061, 4.999999999999992006 ) ) ;
#17807=ADVANCED_FACE ( 'NONE', ( #15531, #1527 ), #15389, .F. ) ;
#17815=CARTESIAN_POINT ( 'NONE',  ( 3.469446951953614189E-15, 40.00000000000000000, 4.999999999999992006 ) ) ;
#17817=CARTESIAN_POINT ( 'NONE',  ( -3.999999999999997335, 28.86250000000000071, 11.30940107675849404 ) ) ;
#17818=LINE ( 'NONE', #13637, #3474 ) ;
#17831=ORIENTED_EDGE ( 'NONE', *, *, #3855, .F. ) ;
#17852=( BOUNDED_CURVE ( )  B_SPLINE_CURVE ( 2, ( #13130, #20711, #21100, #2790, #22808, #24769, #3178, #12857, #20834 ),
 .UNSPECIFIED., .F., .F. ) 
 B_SPLINE_CURVE_WITH_KNOTS ( ( 3, 2, 2, 2, 3 ),
 ( 0.6250000000000000000, 0.6333333333333333037, 0.6500000000000000222, 0.6666666666666666297, 0.6750000000000000444 ),
 .UNSPECIFIED. ) 
 CURVE ( )  GEOMETRIC_REPRESENTATION_ITEM ( )  RATIONAL_B_SPLINE_CURVE ( ( 0.9330127018922194093, 0.9330127018922194093, 1.000000000000000000, 0.8660254037844387076, 1.000000000000000000, 0.8660254037844387076, 1.000000000000000000, 0.9330127018922189652, 0.9330127018922194093 ) ) 
 REPRESENTATION_ITEM ( '' )  );
#17858=CARTESIAN_POINT ( 'NONE',  ( 4.000000000000003553, 28.15000000000000213, 8.999999999999992895 ) ) ;
#17865=CARTESIAN_POINT ( 'NONE',  ( -3.999999999999997335, 26.55624999877096926, 11.30940107675849404 ) ) ;
#17869=CARTESIAN_POINT ( 'NONE',  ( 3.756430356250003655, 28.40312499938548640, 8.999999999999992895 ) ) ;
#17877=EDGE_CURVE ( 'NONE', #1168, #12422, #613, .T. ) ;
#17891=CARTESIAN_POINT ( 'NONE',  ( 2.672651547586948120E-15, 26.49062499938548143, 13.33755215474602984 ) ) ;
#17970=CARTESIAN_POINT ( 'NONE',  ( 1.878215178125000939, 29.67812499938548498, 12.25316411605952283 ) ) ;
#17978=CARTESIAN_POINT ( 'NONE',  ( 3.756430356250004099, 26.07812499938548356, 6.831223922626973533 ) ) ;
#17986=MECHANICAL_DESIGN_GEOMETRIC_PRESENTATION_REPRESENTATION('',(#15485),#4201);
#18001=CARTESIAN_POINT ( 'NONE',  ( -3.999999999999997335, 28.35624999877096997, 11.30940107675849404 ) ) ;
#18006=CARTESIAN_POINT ( 'NONE',  ( -1.878215178124998497, 28.25312499938548427, 12.25316411605951927 ) ) ;
#18034=CARTESIAN_POINT ( 'NONE',  ( 3.735045420075836212E-15, 27.61562499938548498, 4.662447845253954171 ) ) ;
#18061=EDGE_CURVE ( 'NONE', #1665, #18613, #3158, .T. ) ;
#18066=DIRECTION ( 'NONE',  ( 0.000000000000000000, 0.000000000000000000, 1.000000000000000000 ) ) ;
#18068=CARTESIAN_POINT ( 'NONE',  ( 3.878215178125003604, 25.07031249969274356, 8.999999999999992895 ) ) ;
#18072=CARTESIAN_POINT ( 'NONE',  ( 3.834746474454188013E-15, 27.81249999999999645, 4.999999999999992006 ) ) ;
#18085=CARTESIAN_POINT ( 'NONE',  ( 4.000000000000003553, 25.39374999877096784, 8.999999999999992895 ) ) ;
#18088=CARTESIAN_POINT ( 'NONE',  ( 4.000000000000003553, 29.08750000000000213, 6.690598923241489970 ) ) ;
#18122=CARTESIAN_POINT ( 'NONE',  ( 3.756430356250003655, 27.84062499938548640, 8.999999999999992895 ) ) ;
#18124=DIRECTION ( 'NONE',  ( 0.000000000000000000, 0.000000000000000000, -1.000000000000000000 ) ) ;
#18130=CARTESIAN_POINT ( 'NONE',  ( 1.626862140677534194E-14, 27.58750000000000213, 12.99999999999999289 ) ) ;
#18140=CARTESIAN_POINT ( 'NONE',  ( 2.620986760973688460E-15, 27.08124999877096784, 13.61880215351699874 ) ) ;
#18145=CARTESIAN_POINT ( 'NONE',  ( 3.756430356250003655, 28.85312499938548569, 8.999999999999992895 ) ) ;
#18148=CARTESIAN_POINT ( 'NONE',  ( -3.999999999999995559, 27.83124999877096784, 6.690598923241487306 ) ) ;
#18154=CARTESIAN_POINT ( 'NONE',  ( -3.137519842735244810E-15, 27.30624999877096926, 4.999999999999991118 ) ) ;
#18165=CARTESIAN_POINT ( 'NONE',  ( 1.878215178125000939, 29.22812499938548569, 12.25316411605952283 ) ) ;
#18167=LINE ( 'NONE', #4026, #19569 ) ;
#18187=CARTESIAN_POINT ( 'NONE',  ( 3.756430356250003655, 26.49062499938548498, 8.999999999999992895 ) ) ;
#18209=CARTESIAN_POINT ( 'NONE',  ( -3.999999999999997335, 29.31250000000000000, 11.30940107675849404 ) ) ;
#18223=EDGE_LOOP ( 'NONE', ( #23539, #5036, #8948, #8029 ) ) ;
#18235=CARTESIAN_POINT ( 'NONE',  ( 2.672651547586948120E-15, 26.37812499938548427, 13.33755215474602984 ) ) ;
#18248=CARTESIAN_POINT ( 'NONE',  ( 3.959305671612554781E-15, 34.00000000000000000, 12.99999999999999289 ) ) ;
#18251=CARTESIAN_POINT ( 'NONE',  ( 2.620986760973688460E-15, 26.63124999877097565, 13.61880215351699874 ) ) ;
#18279=CARTESIAN_POINT ( 'NONE',  ( 3.756430356250002323, 26.00312499938548427, 11.16877607737301226 ) ) ;
#18294=CARTESIAN_POINT ( 'NONE',  ( -1.071796769724490117, 26.87634618820330701, 4.999999999999992895 ) ) ;
#18304=CARTESIAN_POINT ( 'NONE',  ( 3.756430356250003211, 27.42812499938548143, 6.831223922626973533 ) ) ;
#18352=ORIENTED_EDGE ( 'NONE', *, *, #20348, .T. ) ;
#18359=CARTESIAN_POINT ( 'NONE',  ( 3.756430356250003655, 27.39062499938548356, 8.999999999999992895 ) ) ;
#18360=CARTESIAN_POINT ( 'NONE',  ( 3.469446951953614189E-15, 34.00000000000000000, 8.999999999999992895 ) ) ;
#18377=CARTESIAN_POINT ( 'NONE',  ( 3.756430356250002323, 25.66562499938548569, 11.16877607737301226 ) ) ;
#18407=CARTESIAN_POINT ( 'NONE',  ( -3.756430356249995661, 26.22812499938548214, 6.831223922626973533 ) ) ;
#18412=DIRECTION ( 'NONE',  ( 0.000000000000000000, 1.000000000000000000, 0.000000000000000000 ) ) ;
#18440=CARTESIAN_POINT ( 'NONE',  ( -3.756430356249996105, 26.22812499938548214, 6.831223922626973533 ) ) ;
#18454=CARTESIAN_POINT ( 'NONE',  ( 3.756430356250003655, 25.19687499938548569, 8.999999999999992895 ) ) ;
#18460=VERTEX_POINT ( 'NONE', #18576 ) ;
#18482=CARTESIAN_POINT ( 'NONE',  ( 3.469446951953614189E-15, 40.00000000000000000, 4.999999999999992006 ) ) ;
#18503=CARTESIAN_POINT ( 'NONE',  ( -1.878215178124998497, 26.34062499938548285, 12.25316411605951927 ) ) ;
#18520=CARTESIAN_POINT ( 'NONE',  ( 3.756430356250004099, 26.19062499938548783, 6.831223922626973533 ) ) ;
#18548=CARTESIAN_POINT ( 'NONE',  ( 3.756430356250004099, 29.34062499938548640, 6.831223922626973533 ) ) ;
#18574=CARTESIAN_POINT ( 'NONE',  ( 3.756430356250003211, 25.62812499938548072, 6.831223922626973533 ) ) ;
#18576=CARTESIAN_POINT ( 'NONE',  ( 4.000000000000003553, 25.39374999877096784, 8.999999999999992895 ) ) ;
#18596=LINE ( 'NONE', #20553, #9191 ) ;
#18613=VERTEX_POINT ( 'NONE', #13465 ) ;
#18623=CARTESIAN_POINT ( 'NONE',  ( 3.752267015613588906E-15, 25.11250000000000071, 4.381197846482986158 ) ) ;
#18632=CARTESIAN_POINT ( 'NONE',  ( 3.469446951953614189E-15, 25.00000000000000000, 8.999999999999992895 ) ) ;
#18640=CARTESIAN_POINT ( 'NONE',  ( 2.672651547586948120E-15, 26.49062499938548143, 13.33755215474602984 ) ) ;
#18662=CARTESIAN_POINT ( 'NONE',  ( 2.672651547586948120E-15, 29.19062499938548783, 13.33755215474602984 ) ) ;
#18687=CARTESIAN_POINT ( 'NONE',  ( -3.756430356249997438, 29.00312499938548072, 11.16877607737301048 ) ) ;
#18733=VERTEX_POINT ( 'NONE', #4145 ) ;
#18743=CARTESIAN_POINT ( 'NONE',  ( 4.000000000000003553, 25.03749999999999787, 6.690598923241489970 ) ) ;
#18756=CARTESIAN_POINT ( 'NONE',  ( 3.369928719974892281E-15, 25.50624999877096855, 4.999999999999992006 ) ) ;
#18761=CARTESIAN_POINT ( 'NONE',  ( 1.878215178125004048, 26.22812499938548569, 5.746835883940462963 ) ) ;
#18784=DIRECTION ( 'NONE',  ( -0.000000000000000000, -1.000000000000000000, -0.000000000000000000 ) ) ;
#18785=CARTESIAN_POINT ( 'NONE',  ( 3.469446951953614189E-15, 34.00000000000000000, 3.499999999999992895 ) ) ;
#18793=CARTESIAN_POINT ( 'NONE',  ( -1.878215178124998497, 27.69062499938548427, 12.25316411605951927 ) ) ;
#18825=CARTESIAN_POINT ( 'NONE',  ( 2.672651547586948120E-15, 29.52812499938548285, 13.33755215474603162 ) ) ;
#18831=CARTESIAN_POINT ( 'NONE',  ( 3.756430356250002323, 26.11562499938548498, 11.16877607737301226 ) ) ;
#18836=EDGE_LOOP ( 'NONE', ( #12236, #17831, #4621, #10991 ) ) ;
#18853=AXIS2_PLACEMENT_3D ( 'NONE', #20310, #14708, #12742 ) ;
#18858=VECTOR ( 'NONE', #9528, 1000.000000000000000 ) ;
#18874=ORIENTED_EDGE ( 'NONE', *, *, #6339, .F. ) ;
#18884=CARTESIAN_POINT ( 'NONE',  ( -3.756430356249996994, 29.41562499938548569, 8.999999999999992895 ) ) ;
#18887=CARTESIAN_POINT ( 'NONE',  ( -1.071796769724490117, 26.48259618943233562, 4.999999999999992895 ) ) ;
#18892=( BOUNDED_CURVE ( )  B_SPLINE_CURVE ( 2, ( #5396, #9335, #10888, #19389, #13000, #19126, #20980, #5273, #1359 ),
 .UNSPECIFIED., .F., .F. ) 
 B_SPLINE_CURVE_WITH_KNOTS ( ( 3, 2, 2, 2, 3 ),
 ( 0.2750000000000000222, 0.2833333333333333259, 0.2999999999999999889, 0.3166666666666666519, 0.3250000000000000111 ),
 .UNSPECIFIED. ) 
 CURVE ( )  GEOMETRIC_REPRESENTATION_ITEM ( )  RATIONAL_B_SPLINE_CURVE ( ( 0.9330127018922194093, 0.9330127018922196314, 1.000000000000000000, 0.8660254037844387076, 1.000000000000000000, 0.8660254037844387076, 1.000000000000000000, 0.9330127018922191873, 0.9330127018922194093 ) ) 
 REPRESENTATION_ITEM ( '' )  );
#18903=CARTESIAN_POINT ( 'NONE',  ( 2.620986760973688460E-15, 29.33124999877096784, 13.61880215351699874 ) ) ;
#18930=CARTESIAN_POINT ( 'NONE',  ( -1.878215178124995832, 28.89062499938548356, 5.746835883940462963 ) ) ;
#18936=CARTESIAN_POINT ( 'NONE',  ( -1.999999999999998224, 28.90000000000000213, 12.46410161513774639 ) ) ;
#18942=( BOUNDED_CURVE ( )  B_SPLINE_CURVE ( 2, ( #24898, #18887, #7364, #1482, #1219, #14956, #14836, #11145, #3059 ),
 .UNSPECIFIED., .F., .F. ) 
 B_SPLINE_CURVE_WITH_KNOTS ( ( 3, 2, 2, 2, 3 ),
 ( 0.3250000000000000111, 0.3333333333333333148, 0.3499999999999999778, 0.3666666666666666408, 0.3750000000000000000 ),
 .UNSPECIFIED. ) 
 CURVE ( )  GEOMETRIC_REPRESENTATION_ITEM ( )  RATIONAL_B_SPLINE_CURVE ( ( 0.9330127018922194093, 0.9330127018922196314, 1.000000000000000000, 0.8660254037844387076, 1.000000000000000000, 0.8660254037844387076, 1.000000000000000000, 0.9330127018922194093, 0.9330127018922194093 ) ) 
 REPRESENTATION_ITEM ( '' )  );
#18955=CARTESIAN_POINT ( 'NONE',  ( -1.878215178124995832, 28.89062499938548356, 5.746835883940462963 ) ) ;
#19006=CARTESIAN_POINT ( 'NONE',  ( 1.878215178125004048, 28.81562499938548427, 5.746835883940462963 ) ) ;
#19021=CARTESIAN_POINT ( 'NONE',  ( 3.756430356250004099, 26.64062499938549067, 6.831223922626973533 ) ) ;
#19025=VERTEX_POINT ( 'NONE', #9700 ) ;
#19027=CARTESIAN_POINT ( 'NONE',  ( 3.469446951953614189E-15, 40.00000000000000000, 8.999999999999992895 ) ) ;
#19045=CARTESIAN_POINT ( 'NONE',  ( 3.756430356250003655, 27.39062499938548356, 8.999999999999992895 ) ) ;
#19055=CARTESIAN_POINT ( 'NONE',  ( -3.756430356249996105, 25.89062499938548356, 6.831223922626973533 ) ) ;
#19073=CARTESIAN_POINT ( 'NONE',  ( -1.878215178124995832, 29.34062499938548285, 5.746835883940462963 ) ) ;
#19079=( BOUNDED_CURVE ( )  B_SPLINE_CURVE ( 2, ( #8128, #21592, #23948, #10200, #21982, #4057, #23681, #20144, #9703 ),
 .UNSPECIFIED., .F., .F. ) 
 B_SPLINE_CURVE_WITH_KNOTS ( ( 3, 2, 2, 2, 3 ),
 ( 0.7750000000000000222, 0.7833333333333333259, 0.8000000000000000444, 0.8166666666666666519, 0.8250000000000000666 ),
 .UNSPECIFIED. ) 
 CURVE ( )  GEOMETRIC_REPRESENTATION_ITEM ( )  RATIONAL_B_SPLINE_CURVE ( ( 0.9330127018922194093, 0.9330127018922194093, 1.000000000000000000, 0.8660254037844387076, 1.000000000000000000, 0.8660254037844387076, 1.000000000000000000, 0.9330127018922189652, 0.9330127018922194093 ) ) 
 REPRESENTATION_ITEM ( '' )  );
#19080=CARTESIAN_POINT ( 'NONE',  ( -3.756430356249995661, 26.34062499938548285, 6.831223922626973533 ) ) ;
#19083=CARTESIAN_POINT ( 'NONE',  ( 3.469446951953614189E-15, 40.00000000000000000, 4.999999999999992006 ) ) ;
#19120=ORIENTED_EDGE ( 'NONE', *, *, #10621, .F. ) ;
#19122=CARTESIAN_POINT ( 'NONE',  ( -1.878215178124998497, 29.49062499938548498, 12.25316411605951927 ) ) ;
#19126=CARTESIAN_POINT ( 'NONE',  ( 4.000000000000003553, 26.38750000000000284, 6.690598923241489970 ) ) ;
#19135=ORIENTED_EDGE ( 'NONE', *, *, #21074, .F. ) ;
#19142=CARTESIAN_POINT ( 'NONE',  ( 2.672651547586948120E-15, 26.94062499938548783, 13.33755215474602984 ) ) ;
#19168=CARTESIAN_POINT ( 'NONE',  ( -3.756430356249995661, 27.12812499938548427, 6.831223922626973533 ) ) ;
#19175=ORIENTED_EDGE ( 'NONE', *, *, #3594, .F. ) ;
#19176=CARTESIAN_POINT ( 'NONE',  ( 3.756430356250002323, 25.66562499938548569, 11.16877607737301403 ) ) ;
#19208=CARTESIAN_POINT ( 'NONE',  ( 2.000000000000000888, 27.17500000000000071, 12.46410161513774817 ) ) ;
#19211=CYLINDRICAL_SURFACE ( 'NONE', #15012, 4.000000000000000000 ) ;
#19256=CARTESIAN_POINT ( 'NONE',  ( 3.752267015613588906E-15, 26.91250000000000142, 4.381197846482986158 ) ) ;
#19277=CARTESIAN_POINT ( 'NONE',  ( -3.756430356249996994, 27.72812499938548569, 8.999999999999992895 ) ) ;
#19305=CARTESIAN_POINT ( 'NONE',  ( 3.735045420075836212E-15, 28.40312499938548640, 4.662447845253954171 ) ) ;
#19312=CARTESIAN_POINT ( 'NONE',  ( 2.620986760973688460E-15, 25.73124999877096997, 13.61880215351699874 ) ) ;
#19317=CARTESIAN_POINT ( 'NONE',  ( 2.672651547586948120E-15, 26.94062499938548783, 13.33755215474603162 ) ) ;
#19341=CARTESIAN_POINT ( 'NONE',  ( 1.878215178125004048, 25.32812499938548356, 5.746835883940462963 ) ) ;
#19383=CARTESIAN_POINT ( 'NONE',  ( 4.000000000000003553, 26.80000000000000071, 8.999999999999992895 ) ) ;
#19387=CARTESIAN_POINT ( 'NONE',  ( 2.000000000000000888, 28.07500000000000284, 12.46410161513774817 ) ) ;
#19389=CARTESIAN_POINT ( 'NONE',  ( 4.000000000000001776, 26.31250000000000000, 11.30940107675849760 ) ) ;
#19400=ORIENTED_EDGE ( 'NONE', *, *, #10621, .T. ) ;
#19406=CARTESIAN_POINT ( 'NONE',  ( 1.878215178125000939, 26.97812499938548569, 12.25316411605952283 ) ) ;
#19407=CARTESIAN_POINT ( 'NONE',  ( 2.000000000000003997, 28.16874999877096997, 5.535898384862238508 ) ) ;
#19413=CARTESIAN_POINT ( 'NONE',  ( 3.756430356250004099, 25.62812499938548072, 6.831223922626973533 ) ) ;
#19429=CARTESIAN_POINT ( 'NONE',  ( 1.878215178125000939, 29.56562499938548427, 12.25316411605952283 ) ) ;
#19436=DIRECTION ( 'NONE',  ( 0.000000000000000000, -0.000000000000000000, 1.000000000000000000 ) ) ;
#19438=CARTESIAN_POINT ( 'NONE',  ( 1.878215178125004048, 25.77812499938548640, 5.746835883940462963 ) ) ;
#19448=( BOUNDED_CURVE ( )  B_SPLINE_CURVE ( 2, ( #6872, #22828, #6353, #4509, #14346, #22308, #20733, #22707, #20460 ),
 .UNSPECIFIED., .F., .F. ) 
 B_SPLINE_CURVE_WITH_KNOTS ( ( 3, 2, 2, 2, 3 ),
 ( 0.7249999999999999778, 0.7333333333333332815, 0.7500000000000000000, 0.7666666666666667185, 0.7750000000000000222 ),
 .UNSPECIFIED. ) 
 CURVE ( )  GEOMETRIC_REPRESENTATION_ITEM ( )  RATIONAL_B_SPLINE_CURVE ( ( 0.9330127018922194093, 0.9330127018922194093, 1.000000000000000000, 0.8660254037844387076, 1.000000000000000000, 0.8660254037844387076, 1.000000000000000000, 0.9330127018922194093, 0.9330127018922194093 ) ) 
 REPRESENTATION_ITEM ( '' )  );
#19462=CARTESIAN_POINT ( 'NONE',  ( -3.756430356249996994, 28.62812499938548427, 8.999999999999992895 ) ) ;
#19492=CARTESIAN_POINT ( 'NONE',  ( 3.834746474454188013E-15, 28.20624999877096428, 4.999999999999992006 ) ) ;
#19502=ORIENTED_EDGE ( 'NONE', *, *, #2772, .F. ) ;
#19503=CARTESIAN_POINT ( 'NONE',  ( 2.620986760973688460E-15, 27.13750000000000284, 13.61880215351699874 ) ) ;
#19512=CARTESIAN_POINT ( 'NONE',  ( 4.000000000000003553, 25.93750000000000000, 6.690598923241489970 ) ) ;
#19520=CARTESIAN_POINT ( 'NONE',  ( 1.878215178125004048, 28.02812499938548640, 5.746835883940462963 ) ) ;
#19536=DIRECTION ( 'NONE',  ( -0.000000000000000000, -1.000000000000000000, -0.000000000000000000 ) ) ;
#19551=CARTESIAN_POINT ( 'NONE',  ( -3.999999999999996003, 26.03124999877097068, 6.690598923241487306 ) ) ;
#19556=CARTESIAN_POINT ( 'NONE',  ( -1.878215178124998497, 25.55312499938548854, 12.25316411605951927 ) ) ;
#19557=EDGE_CURVE ( 'NONE', #8387, #18460, #18167, .T. ) ;
#19561=ORIENTED_EDGE ( 'NONE', *, *, #21132, .T. ) ;
#19569=VECTOR ( 'NONE', #24035, 1000.000000000000000 ) ;
#19576=CARTESIAN_POINT ( 'NONE',  ( 4.000000000000003553, 25.84374999877096712, 8.999999999999992895 ) ) ;
#19582=CARTESIAN_POINT ( 'NONE',  ( 1.878215178125000939, 28.77812499938548640, 12.25316411605952283 ) ) ;
#19604=( BOUNDED_CURVE ( )  B_SPLINE_CURVE ( 2, ( #9494, #9382, #23621, #25072, #15655, #15529, #11329, #9252, #17609 ),
 .UNSPECIFIED., .F., .F. ) 
 B_SPLINE_CURVE_WITH_KNOTS ( ( 3, 2, 2, 2, 3 ),
 ( 0.2750000000000000222, 0.2833333333333333259, 0.2999999999999999889, 0.3166666666666666519, 0.3250000000000000111 ),
 .UNSPECIFIED. ) 
 CURVE ( )  GEOMETRIC_REPRESENTATION_ITEM ( )  RATIONAL_B_SPLINE_CURVE ( ( 0.9330127018922194093, 0.9330127018922196314, 1.000000000000000000, 0.8660254037844387076, 1.000000000000000000, 0.8660254037844387076, 1.000000000000000000, 0.9330127018922191873, 0.9330127018922194093 ) ) 
 REPRESENTATION_ITEM ( '' )  );
#19614=DIRECTION ( 'NONE',  ( 0.000000000000000000, 1.000000000000000000, 0.000000000000000000 ) ) ;
#19622=FACE_OUTER_BOUND ( 'NONE', #13008, .T. ) ;
#19623=ORIENTED_EDGE ( 'NONE', *, *, #25197, .F. ) ;
#19637=CARTESIAN_POINT ( 'NONE',  ( 2.620986760973688460E-15, 26.68750000000000000, 13.61880215351699874 ) ) ;
#19642=DIRECTION ( 'NONE',  ( 0.000000000000000000, 0.000000000000000000, -1.000000000000000000 ) ) ;
#19650=CARTESIAN_POINT ( 'NONE',  ( 1.859271017917182139E-15, 29.38749999999999929, 12.99999999999999289 ) ) ;
#19659=CARTESIAN_POINT ( 'NONE',  ( 3.735045420075836212E-15, 29.41562499938548569, 4.662447845253954171 ) ) ;
#19660=CARTESIAN_POINT ( 'NONE',  ( 3.834746474454188013E-15, 28.20624999877096428, 4.999999999999992006 ) ) ;
#19665=ADVANCED_FACE ( 'NONE', ( #11992 ), #22598, .T. ) ;
#19669=CARTESIAN_POINT ( 'NONE',  ( 3.756430356250004099, 25.17812499938548498, 6.831223922626973533 ) ) ;
#19671=AXIS2_PLACEMENT_3D ( 'NONE', #7519, #19536, #17085 ) ;
#19696=CARTESIAN_POINT ( 'NONE',  ( 1.071796769724492338, 29.40759618943233278, 12.99999999999999467 ) ) ;
#19697=ORIENTED_EDGE ( 'NONE', *, *, #1907, .T. ) ;
#19698=CARTESIAN_POINT ( 'NONE',  ( -1.878215178124995832, 27.65312499938548640, 5.746835883940462963 ) ) ;
#19726=CARTESIAN_POINT ( 'NONE',  ( -3.756430356249995661, 27.24062499938548498, 6.831223922626973533 ) ) ;
#19728=CARTESIAN_POINT ( 'NONE',  ( 3.469446951953614189E-15, 40.00000000000000000, 8.999999999999992895 ) ) ;
#19733=DIRECTION ( 'NONE',  ( 0.000000000000000000, 0.000000000000000000, -1.000000000000000000 ) ) ;
#19741=FACE_OUTER_BOUND ( 'NONE', #13858, .T. ) ;
#19752=DIRECTION ( 'NONE',  ( 0.000000000000000000, 0.000000000000000000, 1.000000000000000000 ) ) ;
#19765=CYLINDRICAL_SURFACE ( 'NONE', #6235, 5.500000000000000000 ) ;
#19776=CARTESIAN_POINT ( 'NONE',  ( 4.000000000000001776, 26.31250000000000000, 11.30940107675849760 ) ) ;
#19792=CARTESIAN_POINT ( 'NONE',  ( -1.999999999999998224, 26.14374999877096784, 12.46410161513774639 ) ) ;
#19806=CARTESIAN_POINT ( 'NONE',  ( -1.999999999999998224, 27.55000000000000071, 12.46410161513774639 ) ) ;
#19812=CARTESIAN_POINT ( 'NONE',  ( 3.469446951953614189E-15, 40.00000000000000000, 8.999999999999992895 ) ) ;
#19817=CARTESIAN_POINT ( 'NONE',  ( 4.000000000000003553, 28.09374999877097068, 8.999999999999992895 ) ) ;
#19820=VERTEX_POINT ( 'NONE', #721 ) ;
#19821=CARTESIAN_POINT ( 'NONE',  ( 3.756430356250003655, 27.50312499938548427, 8.999999999999992895 ) ) ;
#19830=CARTESIAN_POINT ( 'NONE',  ( -1.999999999999998224, 27.49374999877096926, 12.46410161513774639 ) ) ;
#19833=LINE ( 'NONE', #25728, #9636 ) ;
#19842=CARTESIAN_POINT ( 'NONE',  ( 3.756430356250003655, 27.95312499938548711, 8.999999999999992895 ) ) ;
#19843=DIRECTION ( 'NONE',  ( -0.000000000000000000, -1.000000000000000000, -0.000000000000000000 ) ) ;
#19849=CARTESIAN_POINT ( 'NONE',  ( 3.469446951953614189E-15, 40.00000000000000000, 8.999999999999992895 ) ) ;
#19865=FACE_OUTER_BOUND ( 'NONE', #22770, .T. ) ;
#19870=FACE_OUTER_BOUND ( 'NONE', #25240, .T. ) ;
#19880=EDGE_LOOP ( 'NONE', ( #1478, #15917, #12273, #9416, #3968, #1702, #22854, #15595 ) ) ;
#19886=CARTESIAN_POINT ( 'NONE',  ( 2.000000000000003997, 25.46874999877096712, 5.535898384862238508 ) ) ;
#19889=CARTESIAN_POINT ( 'NONE',  ( 2.000000000000000888, 28.97500000000000142, 12.46410161513774817 ) ) ;
#19909=CARTESIAN_POINT ( 'NONE',  ( -3.756430356249996994, 29.07812499938548356, 8.999999999999992895 ) ) ;
#19914=ORIENTED_EDGE ( 'NONE', *, *, #20242, .F. ) ;
#19916=CARTESIAN_POINT ( 'NONE',  ( -3.756430356249995661, 26.22812499938548214, 6.831223922626973533 ) ) ;
#19935=CARTESIAN_POINT ( 'NONE',  ( -3.999999999999996003, 27.83124999877096784, 6.690598923241487306 ) ) ;
#19940=CARTESIAN_POINT ( 'NONE',  ( -1.878215178124998497, 27.35312499938548569, 12.25316411605951927 ) ) ;
#19964=CARTESIAN_POINT ( 'NONE',  ( 1.878215178125004048, 28.02812499938548640, 5.746835883940462963 ) ) ;
#19975=ORIENTED_EDGE ( 'NONE', *, *, #23543, .F. ) ;
#19992=CARTESIAN_POINT ( 'NONE',  ( -3.756430356249997438, 26.75312499938548427, 11.16877607737301048 ) ) ;
#20025=EDGE_CURVE ( 'NONE', #21478, #13240, #25788, .T. ) ;
#20041=ORIENTED_EDGE ( 'NONE', *, *, #9608, .F. ) ;
#20050=CARTESIAN_POINT ( 'NONE',  ( 3.735045420075836212E-15, 27.95312499938548001, 4.662447845253954171 ) ) ;
#20074=CARTESIAN_POINT ( 'NONE',  ( -3.999999999999996003, 28.28124999877096712, 6.690598923241487306 ) ) ;
#20078=CARTESIAN_POINT ( 'NONE',  ( 3.756430356250002323, 28.36562499938548854, 11.16877607737301403 ) ) ;
#20089=VECTOR ( 'NONE', #20414, 999.9999999999998863 ) ;
#20104=CARTESIAN_POINT ( 'NONE',  ( 3.756430356250004099, 25.62812499938548072, 6.831223922626973533 ) ) ;
#20113=CYLINDRICAL_SURFACE ( 'NONE', #2473, 4.000000000000000000 ) ;
#20123=CARTESIAN_POINT ( 'NONE',  ( -1.999999999999998224, 26.59374999877096712, 12.46410161513774639 ) ) ;
#20132=CARTESIAN_POINT ( 'NONE',  ( 2.672651547586948120E-15, 26.82812499938548356, 13.33755215474603162 ) ) ;
#20144=CARTESIAN_POINT ( 'NONE',  ( 1.071796769724487675, 28.69240381056766509, 4.999999999999988454 ) ) ;
#20155=CARTESIAN_POINT ( 'NONE',  ( 4.000000000000003553, 28.60000000000000142, 8.999999999999992895 ) ) ;
#20173=EDGE_CURVE ( 'NONE', #19025, #3732, #6080, .T. ) ;
#20184=CARTESIAN_POINT ( 'NONE',  ( -3.756430356249997882, 28.10312499938548569, 11.16877607737301226 ) ) ;
#20191=CARTESIAN_POINT ( 'NONE',  ( -1.071796769724485454, 26.21740381056766367, 12.99999999999999467 ) ) ;
#20199=EDGE_LOOP ( 'NONE', ( #2338, #18874, #25809, #7289 ) ) ;
#20200=CARTESIAN_POINT ( 'NONE',  ( -3.999999999999996003, 27.38124999877096855, 6.690598923241487306 ) ) ;
#20205=CARTESIAN_POINT ( 'NONE',  ( 1.878215178125000939, 27.42812499938548498, 12.25316411605952283 ) ) ;
#20231=CARTESIAN_POINT ( 'NONE',  ( 3.756430356250003655, 29.30312499938548498, 8.999999999999992895 ) ) ;
#20242=EDGE_CURVE ( 'NONE', #11825, #5668, #7245, .T. ) ;
#20252=FILL_AREA_STYLE ('',( #10059 ) ) ;
#20257=CARTESIAN_POINT ( 'NONE',  ( -3.756430356249996994, 26.71562499938548285, 8.999999999999992895 ) ) ;
#20273=EDGE_LOOP ( 'NONE', ( #21281, #23052, #20900, #25719 ) ) ;
#20307=CARTESIAN_POINT ( 'NONE',  ( -1.878215178124995832, 26.64062499938548711, 5.746835883940462963 ) ) ;
#20310=CARTESIAN_POINT ( 'NONE',  ( 3.469446951953614189E-15, 40.00000000000000000, 8.999999999999992895 ) ) ;
#20316=CARTESIAN_POINT ( 'NONE',  ( -1.999999999999998224, 26.20000000000000284, 12.46410161513774639 ) ) ;
#20325=CARTESIAN_POINT ( 'NONE',  ( 3.752267015613588906E-15, 28.20624999877096784, 4.381197846482986158 ) ) ;
#20332=CARTESIAN_POINT ( 'NONE',  ( 1.626862140677534194E-14, 27.98124999877096997, 12.99999999999999289 ) ) ;
#20333=ORIENTED_EDGE ( 'NONE', *, *, #9266, .F. ) ;
#20334=EDGE_LOOP ( 'NONE', ( #5803, #17445, #21320, #14660 ) ) ;
#20348=EDGE_CURVE ( 'NONE', #8387, #24266, #9894, .T. ) ;
#20351=CARTESIAN_POINT ( 'NONE',  ( 3.756430356250003655, 26.49062499938548498, 8.999999999999992895 ) ) ;
#20377=CARTESIAN_POINT ( 'NONE',  ( -1.878215178124998497, 25.44062499938548427, 12.25316411605951927 ) ) ;
#20384=CARTESIAN_POINT ( 'NONE',  ( 1.626862140677534194E-14, 28.03750000000000497, 12.99999999999999289 ) ) ;
#20412=LINE ( 'NONE', #18482, #23461 ) ;
#20414=DIRECTION ( 'NONE',  ( 0.8660254037844397068, 0.4999999999999983347, -0.000000000000000000 ) ) ;
#20436=CARTESIAN_POINT ( 'NONE',  ( 3.756430356250003655, 26.94062499938548427, 8.999999999999992895 ) ) ;
#20438=VECTOR ( 'NONE', #667, 1000.000000000000000 ) ;
#20455=CARTESIAN_POINT ( 'NONE',  ( 3.756430356250003655, 25.70312499938548356, 8.999999999999992895 ) ) ;
#20460=CARTESIAN_POINT ( 'NONE',  ( 1.859271017917182139E-15, 28.88124999877096499, 12.99999999999999289 ) ) ;
#20464=CARTESIAN_POINT ( 'NONE',  ( -1.999999999999995781, 25.54374999877096997, 5.535898384862237620 ) ) ;
#20475=CYLINDRICAL_SURFACE ( 'NONE', #25462, 4.000000000000000000 ) ;
#20479=AXIS2_PLACEMENT_3D ( 'NONE', #21877, #7490, #15481 ) ;
#20489=CARTESIAN_POINT ( 'NONE',  ( 2.672651547586948120E-15, 26.37812499938548427, 13.33755215474602984 ) ) ;
#20490=AXIS2_PLACEMENT_3D ( 'NONE', #16091, #25760, #19752 ) ;
#20523=CARTESIAN_POINT ( 'NONE',  ( -3.756430356249996105, 26.67812499938548498, 6.831223922626973533 ) ) ;
#20528=SHAPE_REPRESENTATION ( 'dust cap', ( #21036 ), #8945 ) ;
#20553=CARTESIAN_POINT ( 'NONE',  ( 3.959305671612554781E-15, 40.00000000000000000, 12.99999999999999289 ) ) ;
#20581=CARTESIAN_POINT ( 'NONE',  ( 4.000000000000003553, 25.48750000000000071, 6.690598923241489970 ) ) ;
#20599=CARTESIAN_POINT ( 'NONE',  ( 4.000000000000003553, 29.03124999877096712, 6.690598923241489970 ) ) ;
#20627=CARTESIAN_POINT ( 'NONE',  ( -1.878215178124995832, 29.00312499938548427, 5.746835883940462963 ) ) ;
#20642=ORIENTED_EDGE ( 'NONE', *, *, #20801, .T. ) ;
#20657=CARTESIAN_POINT ( 'NONE',  ( 1.878215178125000939, 27.76562499938548356, 12.25316411605952283 ) ) ;
#20664=CARTESIAN_POINT ( 'NONE',  ( 4.000000000000003553, 27.64374999877096784, 8.999999999999992895 ) ) ;
#20699=EDGE_CURVE ( 'NONE', #14520, #5668, #1734, .T. ) ;
#20710=CARTESIAN_POINT ( 'NONE',  ( 2.000000000000003997, 25.97500000000000142, 5.535898384862238508 ) ) ;
#20711=CARTESIAN_POINT ( 'NONE',  ( -1.071796769724487230, 28.22634618820330132, 4.999999999999992006 ) ) ;
#20728=CARTESIAN_POINT ( 'NONE',  ( 4.000000000000003553, 28.99374999877096926, 8.999999999999992895 ) ) ;
#20731=EDGE_LOOP ( 'NONE', ( #9596, #16918, #8218, #22733 ) ) ;
#20733=CARTESIAN_POINT ( 'NONE',  ( -1.999999999999998224, 28.84374999877096712, 12.46410161513774639 ) ) ;
#20734=CYLINDRICAL_SURFACE ( 'NONE', #10055, 4.000000000000000000 ) ;
#20755=CARTESIAN_POINT ( 'NONE',  ( -3.756430356249995661, 27.57812499938548356, 6.831223922626973533 ) ) ;
#20759=ORIENTED_EDGE ( 'NONE', *, *, #14187, .T. ) ;
#20766=( BOUNDED_SURFACE ( )  B_SPLINE_SURFACE ( 1, 2, ( 
 ( #7290, #13297, #21271, #11461, #15149, #1525, #3354, #17097, #23495, #19312, #1407, #17361, #5582, #25586, #5699, #11579, #1793, #19551, #1654, #9630, #7406, #15385, #7670, #13678, #21651, #3733, #11717, #13178, #23117, #21148, #21916, #17865, #334, #18251, #2300, #13947, #6348, #24261, #13813, #23880, #21792, #3874, #24005, #14070, #15907, #18140, #10007, #5965, #90, #22174, #12233, #5827, #6086, #20200, #8308, #22036, #7920, #16044, #2039, #3997, #11964, #12098, #11846, #12359, #4259, #19935, #25711, #23740, #22303, #14341, #4119, #10257, #19817, #16294, #4380, #20325, #9761, #20074, #2176, #18001, #1918, #17740, #7792, #8061, #15771, #9879, #25837, #10137, #214, #8184, #16162, #24125, #6211, #14201, #10907, #8690, #20728, #20599, #8967, #10377, #986, #851, #22564, #4504, #2942, #18903, #16942, #8446, #14583, #24911, #6867, #22822, #6596, #22949, #4646, #6987, #16555, #12628, #2415, #10523, #8832 ),
 ( #14971, #6732, #14724, #5033, #6475, #477, #8574, #14850, #24645, #2806, #4899, #18377, #20455, #24399, #12481, #13016, #12876, #10770, #16435, #2554, #14461, #2685, #16677, #22423, #723, #18520, #18761, #607, #24514, #16820, #10646, #24785, #22702, #18640, #4782, #12756, #20852, #19021, #3582, #7377, #7125, #9216, #17206, #23594, #25177, #19142, #19406, #15112, #11160, #1621, #11040, #25037, #21238, #9594, #1233, #17063, #3459, #7259, #1376, #13149, #1104, #25558, #23086, #7640, #21113, #9079, #19277, #5172, #3192, #15238, #15354, #15627, #23203, #5287, #19520, #21503, #5673, #13264, #20996, #11433, #5418, #15496, #3320, #17581, #11552, #3074, #11295, #9352, #1497, #13402, #23464, #17333, #25299, #23327, #21379, #9470, #17447, #25415, #7504, #5552, #13536, #11939, #19909, #9855, #6183, #2008, #15877, #5936, #24101, #1767, #7888, #19659, #25684, #3843, #14172, #13652, #6063, #16140, #17970, #21891, #4090 ) ),
 .UNSPECIFIED., .F., .F., .F. ) 
 B_SPLINE_SURFACE_WITH_KNOTS ( ( 2, 2 ),
 ( 3, 2, 2, 2, 2, 2, 2, 2, 2, 2, 2, 2, 2, 2, 2, 2, 2, 2, 2, 2, 2, 2, 2, 2, 2, 2, 2, 2, 2, 2, 2, 2, 2, 2, 2, 2, 2, 2, 2, 2, 2, 2, 2, 2, 2, 2, 2, 2, 2, 2, 2, 2, 2, 2, 2, 2, 2, 2, 2, 2, 3 ),
 ( 0.000000000000000000, 1.000000000000000000 ),
 ( 0.000000000000000000, 0.01666666666666666644, 0.03333333333333333287, 0.05000000000000000278, 0.06666666666666666574, 0.08333333333333332871, 0.1000000000000000056, 0.1166666666666666685, 0.1333333333333333315, 0.1499999999999999944, 0.1666666666666666574, 0.1833333333333333204, 0.2000000000000000111, 0.2166666666666666741, 0.2333333333333333370, 0.2500000000000000000, 0.2666666666666666630, 0.2833333333333333259, 0.2999999999999999889, 0.3166666666666666519, 0.3333333333333333148, 0.3499999999999999778, 0.3666666666666666408, 0.3833333333333333592, 0.4000000000000000222, 0.4166666666666666852, 0.4333333333333333481, 0.4500000000000000111, 0.4666666666666666741, 0.4833333333333333370, 0.5000000000000000000, 0.5166666666666667185, 0.5333333333333333259, 0.5500000000000000444, 0.5666666666666666519, 0.5833333333333333703, 0.5999999999999999778, 0.6166666666666666963, 0.6333333333333333037, 0.6500000000000000222, 0.6666666666666666297, 0.6833333333333333481, 0.6999999999999999556, 0.7166666666666666741, 0.7333333333333332815, 0.7500000000000000000, 0.7666666666666667185, 0.7833333333333333259, 0.8000000000000000444, 0.8166666666666666519, 0.8333333333333333703, 0.8499999999999999778, 0.8666666666666666963, 0.8833333333333333037, 0.9000000000000000222, 0.9166666666666666297, 0.9333333333333333481, 0.9499999999999999556, 0.9666666666666666741, 0.9833333333333332815, 1.000000000000000000 ),
 .UNSPECIFIED. ) 
 GEOMETRIC_REPRESENTATION_ITEM ( )  RATIONAL_B_SPLINE_SURFACE ( (
 ( 1.000000000000000000, 0.8660254037844387076, 1.000000000000000000, 0.8660254037844387076, 1.000000000000000000, 0.8660254037844387076, 1.000000000000000000, 0.8660254037844387076, 1.000000000000000000, 0.8660254037844387076, 1.000000000000000000, 0.8660254037844387076, 1.000000000000000000, 0.8660254037844387076, 1.000000000000000000, 0.8660254037844387076, 1.000000000000000000, 0.8660254037844387076, 1.000000000000000000, 0.8660254037844387076, 1.000000000000000000, 0.8660254037844387076, 1.000000000000000000, 0.8660254037844387076, 1.000000000000000000, 0.8660254037844387076, 1.000000000000000000, 0.8660254037844387076, 1.000000000000000000, 0.8660254037844387076, 1.000000000000000000, 0.8660254037844387076, 1.000000000000000000, 0.8660254037844387076, 1.000000000000000000, 0.8660254037844387076, 1.000000000000000000, 0.8660254037844387076, 1.000000000000000000, 0.8660254037844387076, 1.000000000000000000, 0.8660254037844387076, 1.000000000000000000, 0.8660254037844387076, 1.000000000000000000, 0.8660254037844387076, 1.000000000000000000, 0.8660254037844387076, 1.000000000000000000, 0.8660254037844387076, 1.000000000000000000, 0.8660254037844387076, 1.000000000000000000, 0.8660254037844387076, 1.000000000000000000, 0.8660254037844387076, 1.000000000000000000, 0.8660254037844387076, 1.000000000000000000, 0.8660254037844387076, 1.000000000000000000, 0.8660254037844387076, 1.000000000000000000, 0.8660254037844387076, 1.000000000000000000, 0.8660254037844387076, 1.000000000000000000, 0.8660254037844387076, 1.000000000000000000, 0.8660254037844387076, 1.000000000000000000, 0.8660254037844387076, 1.000000000000000000, 0.8660254037844387076, 1.000000000000000000, 0.8660254037844387076, 1.000000000000000000, 0.8660254037844387076, 1.000000000000000000, 0.8660254037844387076, 1.000000000000000000, 0.8660254037844387076, 1.000000000000000000, 0.8660254037844387076, 1.000000000000000000, 0.8660254037844387076, 1.000000000000000000, 0.8660254037844387076, 1.000000000000000000, 0.8660254037844387076, 1.000000000000000000, 0.8660254037844387076, 1.000000000000000000, 0.8660254037844387076, 1.000000000000000000, 0.8660254037844387076, 1.000000000000000000, 0.8660254037844387076, 1.000000000000000000, 0.8660254037844387076, 1.000000000000000000, 0.8660254037844387076, 1.000000000000000000, 0.8660254037844387076, 1.000000000000000000, 0.8660254037844387076, 1.000000000000000000, 0.8660254037844387076, 1.000000000000000000, 0.8660254037844387076, 1.000000000000000000, 0.8660254037844387076, 1.000000000000000000, 0.8660254037844387076, 1.000000000000000000, 0.8660254037844387076, 1.000000000000000000, 0.8660254037844387076, 1.000000000000000000, 0.8660254037844387076, 1.000000000000000000),
 ( 1.000000000000000000, 0.8660254037844387076, 1.000000000000000000, 0.8660254037844387076, 1.000000000000000000, 0.8660254037844387076, 1.000000000000000000, 0.8660254037844387076, 1.000000000000000000, 0.8660254037844387076, 1.000000000000000000, 0.8660254037844387076, 1.000000000000000000, 0.8660254037844387076, 1.000000000000000000, 0.8660254037844387076, 1.000000000000000000, 0.8660254037844387076, 1.000000000000000000, 0.8660254037844387076, 1.000000000000000000, 0.8660254037844387076, 1.000000000000000000, 0.8660254037844387076, 1.000000000000000000, 0.8660254037844387076, 1.000000000000000000, 0.8660254037844387076, 1.000000000000000000, 0.8660254037844387076, 1.000000000000000000, 0.8660254037844387076, 1.000000000000000000, 0.8660254037844387076, 1.000000000000000000, 0.8660254037844387076, 1.000000000000000000, 0.8660254037844387076, 1.000000000000000000, 0.8660254037844387076, 1.000000000000000000, 0.8660254037844387076, 1.000000000000000000, 0.8660254037844387076, 1.000000000000000000, 0.8660254037844387076, 1.000000000000000000, 0.8660254037844387076, 1.000000000000000000, 0.8660254037844387076, 1.000000000000000000, 0.8660254037844387076, 1.000000000000000000, 0.8660254037844387076, 1.000000000000000000, 0.8660254037844387076, 1.000000000000000000, 0.8660254037844387076, 1.000000000000000000, 0.8660254037844387076, 1.000000000000000000, 0.8660254037844387076, 1.000000000000000000, 0.8660254037844387076, 1.000000000000000000, 0.8660254037844387076, 1.000000000000000000, 0.8660254037844387076, 1.000000000000000000, 0.8660254037844387076, 1.000000000000000000, 0.8660254037844387076, 1.000000000000000000, 0.8660254037844387076, 1.000000000000000000, 0.8660254037844387076, 1.000000000000000000, 0.8660254037844387076, 1.000000000000000000, 0.8660254037844387076, 1.000000000000000000, 0.8660254037844387076, 1.000000000000000000, 0.8660254037844387076, 1.000000000000000000, 0.8660254037844387076, 1.000000000000000000, 0.8660254037844387076, 1.000000000000000000, 0.8660254037844387076, 1.000000000000000000, 0.8660254037844387076, 1.000000000000000000, 0.8660254037844387076, 1.000000000000000000, 0.8660254037844387076, 1.000000000000000000, 0.8660254037844387076, 1.000000000000000000, 0.8660254037844387076, 1.000000000000000000, 0.8660254037844387076, 1.000000000000000000, 0.8660254037844387076, 1.000000000000000000, 0.8660254037844387076, 1.000000000000000000, 0.8660254037844387076, 1.000000000000000000, 0.8660254037844387076, 1.000000000000000000, 0.8660254037844387076, 1.000000000000000000, 0.8660254037844387076, 1.000000000000000000, 0.8660254037844387076, 1.000000000000000000, 0.8660254037844387076, 1.000000000000000000, 0.8660254037844387076, 1.000000000000000000) ) ) 
 REPRESENTATION_ITEM ( '' )  SURFACE ( )  );
#20781=CARTESIAN_POINT ( 'NONE',  ( -3.756430356249997438, 28.10312499938548569, 11.16877607737301048 ) ) ;
#20786=CARTESIAN_POINT ( 'NONE',  ( 3.756430356250004099, 25.74062499938548143, 6.831223922626973533 ) ) ;
#20787=DIRECTION ( 'NONE',  ( 0.000000000000000000, 0.000000000000000000, -1.000000000000000000 ) ) ;
#20792=CARTESIAN_POINT ( 'NONE',  ( 3.469446951953614189E-15, 40.00000000000000000, 8.999999999999992895 ) ) ;
#20801=EDGE_CURVE ( 'NONE', #19820, #14690, #12793, .T. ) ;
#20833=CARTESIAN_POINT ( 'NONE',  ( 4.000000000000003553, 25.44999999999999929, 8.999999999999992895 ) ) ;
#20834=CARTESIAN_POINT ( 'NONE',  ( 1.626862140677534194E-14, 28.43124999877096570, 12.99999999999999289 ) ) ;
#20852=CARTESIAN_POINT ( 'NONE',  ( 3.756430356250003655, 26.60312499938548569, 8.999999999999992895 ) ) ;
#20878=AXIS2_PLACEMENT_3D ( 'NONE', #19849, #25489, #19733 ) ;
#20884=CARTESIAN_POINT ( 'NONE',  ( 1.878215178125004048, 28.81562499938548427, 5.746835883940462963 ) ) ;
#20897=ORIENTED_EDGE ( 'NONE', *, *, #3811, .F. ) ;
#20900=ORIENTED_EDGE ( 'NONE', *, *, #21998, .T. ) ;
#20917=CARTESIAN_POINT ( 'NONE',  ( 3.756430356250003655, 27.84062499938548640, 8.999999999999992895 ) ) ;
#20924=CARTESIAN_POINT ( 'NONE',  ( 3.735045420075836212E-15, 25.36562499938548498, 4.662447845253954171 ) ) ;
#20965=EDGE_CURVE ( 'NONE', #10854, #21434, #3112, .T. ) ;
#20971=VERTEX_POINT ( 'NONE', #15154 ) ;
#20977=CARTESIAN_POINT ( 'NONE',  ( -1.999999999999995781, 25.60000000000000142, 5.535898384862237620 ) ) ;
#20978=CARTESIAN_POINT ( 'NONE',  ( 1.859271017917182139E-15, 27.08124999877096784, 12.99999999999999289 ) ) ;
#20980=CARTESIAN_POINT ( 'NONE',  ( 2.000000000000003997, 26.42500000000000071, 5.535898384862238508 ) ) ;
#20992=EDGE_CURVE ( 'NONE', #5942, #4929, #24952, .T. ) ;
#20996=CARTESIAN_POINT ( 'NONE',  ( -3.756430356249996994, 28.17812499938548498, 8.999999999999992895 ) ) ;
#21023=CARTESIAN_POINT ( 'NONE',  ( -3.756430356249995661, 26.67812499938548498, 6.831223922626973533 ) ) ;
#21036=AXIS2_PLACEMENT_3D ( 'NONE', #13353, #15703, #13223 ) ;
#21051=CARTESIAN_POINT ( 'NONE',  ( 1.878215178125004048, 28.36562499938548143, 5.746835883940462963 ) ) ;
#21056=CARTESIAN_POINT ( 'NONE',  ( -3.756430356249996994, 26.37812499938548783, 8.999999999999992895 ) ) ;
#21074=EDGE_CURVE ( 'NONE', #14690, #21434, #19448, .T. ) ;
#21099=CARTESIAN_POINT ( 'NONE',  ( -3.999999999999997335, 25.71250000000000213, 11.30940107675849404 ) ) ;
#21100=CARTESIAN_POINT ( 'NONE',  ( -1.999999999999995781, 28.24374999877096570, 5.535898384862237620 ) ) ;
#21113=CARTESIAN_POINT ( 'NONE',  ( -1.878215178124995832, 27.65312499938548640, 5.746835883940462963 ) ) ;
#21116=ORIENTED_EDGE ( 'NONE', *, *, #18061, .T. ) ;
#21119=CARTESIAN_POINT ( 'NONE',  ( 3.834746474454188013E-15, 26.40624999877096357, 4.999999999999992006 ) ) ;
#21120=EDGE_LOOP ( 'NONE', ( #14280, #20333, #20897 ) ) ;
#21132=EDGE_CURVE ( 'NONE', #15816, #22942, #22570, .T. ) ;
#21142=CARTESIAN_POINT ( 'NONE',  ( -1.878215178124995832, 27.09062499938548640, 5.746835883940462963 ) ) ;
#21147=AXIS2_PLACEMENT_3D ( 'NONE', #19812, #3993, #17602 ) ;
#21148=CARTESIAN_POINT ( 'NONE',  ( -3.999999999999996003, 26.48124999877096641, 6.690598923241487306 ) ) ;
#21153=CARTESIAN_POINT ( 'NONE',  ( 1.878215178125004048, 25.32812499938548356, 5.746835883940462963 ) ) ;
#21157=ORIENTED_EDGE ( 'NONE', *, *, #2599, .T. ) ;
#21162=CARTESIAN_POINT ( 'NONE',  ( 1.071796769724487675, 29.08615380933863293, 4.999999999999988454 ) ) ;
#21168=CARTESIAN_POINT ( 'NONE',  ( 2.672651547586948120E-15, 28.17812499938548143, 13.33755215474603162 ) ) ;
#21174=CARTESIAN_POINT ( 'NONE',  ( -3.756430356249997882, 25.51562499938548356, 11.16877607737301226 ) ) ;
#21175=CARTESIAN_POINT ( 'NONE',  ( -3.999999999999995559, 29.63124999877096855, 6.690598923241487306 ) ) ;
#21183=ORIENTED_EDGE ( 'NONE', *, *, #24897, .F. ) ;
#21217=CARTESIAN_POINT ( 'NONE',  ( -1.999999999999995781, 27.85000000000000142, 5.535898384862237620 ) ) ;
#21220=CYLINDRICAL_SURFACE ( 'NONE', #8756, 4.000000000000000000 ) ;
#21236=CARTESIAN_POINT ( 'NONE',  ( -3.999999999999995559, 26.98750000000000071, 6.690598923241487306 ) ) ;
#21238=CARTESIAN_POINT ( 'NONE',  ( -1.878215178124995832, 27.20312499938548711, 5.746835883940462963 ) ) ;
#21244=CARTESIAN_POINT ( 'NONE',  ( 5.577813053751546416E-15, 25.73124999877096997, 12.99999999999999289 ) ) ;
#21266=CARTESIAN_POINT ( 'NONE',  ( 3.756430356250003655, 27.84062499938548640, 8.999999999999992895 ) ) ;
#21271=CARTESIAN_POINT ( 'NONE',  ( 2.000000000000003997, 25.46874999877096712, 5.535898384862238508 ) ) ;
#21275=CARTESIAN_POINT ( 'NONE',  ( -3.756430356249996105, 26.79062499938548569, 6.831223922626973533 ) ) ;
#21281=ORIENTED_EDGE ( 'NONE', *, *, #7935, .F. ) ;
#21294=AXIS2_PLACEMENT_3D ( 'NONE', #21581, #19614, #18066 ) ;
#21310=CARTESIAN_POINT ( 'NONE',  ( 3.959305671612554781E-15, 40.00000000000000000, 12.99999999999999289 ) ) ;
#21320=ORIENTED_EDGE ( 'NONE', *, *, #25301, .T. ) ;
#21323=CARTESIAN_POINT ( 'NONE',  ( 3.469446951953614189E-15, 40.00000000000000000, 4.999999999999992006 ) ) ;
#21338=AXIS2_PLACEMENT_3D ( 'NONE', #15860, #17704, #3959 ) ;
#21357=CARTESIAN_POINT ( 'NONE',  ( 2.000000000000000888, 26.27499999999999858, 12.46410161513774817 ) ) ;
#21373=ORIENTED_EDGE ( 'NONE', *, *, #20173, .F. ) ;
#21379=CARTESIAN_POINT ( 'NONE',  ( 1.878215178125000939, 28.77812499938548640, 12.25316411605952283 ) ) ;
#21389=CARTESIAN_POINT ( 'NONE',  ( 3.735045420075836212E-15, 25.25312499938548783, 4.662447845253954171 ) ) ;
#21413=VERTEX_POINT ( 'NONE', #16027 ) ;
#21414=CARTESIAN_POINT ( 'NONE',  ( 3.756430356250003211, 27.09062499938548640, 6.831223922626973533 ) ) ;
#21434=VERTEX_POINT ( 'NONE', #16150 ) ;
#21437=CARTESIAN_POINT ( 'NONE',  ( -3.756430356249995661, 28.59062499938548640, 6.831223922626973533 ) ) ;
#21443=CARTESIAN_POINT ( 'NONE',  ( 3.469446951953614189E-15, 25.00000000000000000, 8.999999999999992895 ) ) ;
#21478=VERTEX_POINT ( 'NONE', #4491 ) ;
#21487=CARTESIAN_POINT ( 'NONE',  ( 4.000000000000003553, 26.83749999999999503, 6.690598923241489970 ) ) ;
#21503=CARTESIAN_POINT ( 'NONE',  ( 3.735045420075836212E-15, 28.06562499938548427, 4.662447845253954171 ) ) ;
#21523=FACE_OUTER_BOUND ( 'NONE', #12658, .T. ) ;
#21532=CARTESIAN_POINT ( 'NONE',  ( -1.878215178124995832, 25.40312499938548640, 5.746835883940462963 ) ) ;
#21556=CARTESIAN_POINT ( 'NONE',  ( -3.756430356249997882, 28.66562499938548569, 11.16877607737301226 ) ) ;
#21564=ORIENTED_EDGE ( 'NONE', *, *, #6324, .F. ) ;
#21581=CARTESIAN_POINT ( 'NONE',  ( 3.469446951953614189E-15, 46.00000000000000000, 8.999999999999992895 ) ) ;
#21591=ORIENTED_EDGE ( 'NONE', *, *, #1365, .T. ) ;
#21592=CARTESIAN_POINT ( 'NONE',  ( 1.071796769724492338, 28.50759618943233775, 12.99999999999999467 ) ) ;
#21605=CARTESIAN_POINT ( 'NONE',  ( -3.999999999999996003, 26.08750000000000213, 6.690598923241487306 ) ) ;
#21612=CARTESIAN_POINT ( 'NONE',  ( -1.071796769724493448, 29.18259618943233136, 4.999999999999995559 ) ) ;
#21621=CARTESIAN_POINT ( 'NONE',  ( 1.626862140677534194E-14, 27.98124999877096997, 12.99999999999999289 ) ) ;
#21632=EDGE_CURVE ( 'NONE', #7170, #16109, #15733, .T. ) ;
#21644=CARTESIAN_POINT ( 'NONE',  ( 3.756430356250004099, 29.22812499938548925, 6.831223922626973533 ) ) ;
#21651=CARTESIAN_POINT ( 'NONE',  ( 4.000000000000003553, 26.29374999877096997, 8.999999999999992895 ) ) ;
#21655=CARTESIAN_POINT ( 'NONE',  ( -3.756430356249996994, 28.62812499938548427, 8.999999999999992895 ) ) ;
#21682=CARTESIAN_POINT ( 'NONE',  ( 3.756430356250002323, 26.56562499938548427, 11.16877607737301226 ) ) ;
#21700=ADVANCED_FACE ( 'NONE', ( #15342 ), #21220, .T. ) ;
#21724=DIRECTION ( 'NONE',  ( -0.000000000000000000, -1.000000000000000000, -0.000000000000000000 ) ) ;
#21726=AXIS2_PLACEMENT_3D ( 'NONE', #13361, #5890, #13616 ) ;
#21736=CARTESIAN_POINT ( 'NONE',  ( -1.999999999999995781, 26.95000000000000284, 5.535898384862237620 ) ) ;
#21738=AXIS2_PLACEMENT_3D ( 'NONE', #10223, #14036, #9969 ) ;
#21759=CARTESIAN_POINT ( 'NONE',  ( -3.999999999999996447, 26.06874999877096855, 8.999999999999992895 ) ) ;
#21786=CARTESIAN_POINT ( 'NONE',  ( 1.071796769724498999, 28.05759618943233491, 12.99999999999998757 ) ) ;
#21792=CARTESIAN_POINT ( 'NONE',  ( -1.999999999999995781, 26.89374999877097139, 5.535898384862237620 ) ) ;
#21796=CARTESIAN_POINT ( 'NONE',  ( 3.735045420075836212E-15, 28.51562499938548356, 4.662447845253954171 ) ) ;
#21802=EDGE_LOOP ( 'NONE', ( #17144, #287, #12851, #23779 ) ) ;
#21822=CARTESIAN_POINT ( 'NONE',  ( -1.878215178124998497, 26.90312499938548285, 12.25316411605951927 ) ) ;
#21844=CARTESIAN_POINT ( 'NONE',  ( 3.878215178125003604, 25.07031249969274356, 8.999999999999992895 ) ) ;
#21845=DIRECTION ( 'NONE',  ( -0.8660254037844397068, 0.4999999999999983347, -0.000000000000000000 ) ) ;
#21859=VERTEX_POINT ( 'NONE', #14153 ) ;
#21871=CARTESIAN_POINT ( 'NONE',  ( 4.000000000000003553, 28.63750000000000284, 6.690598923241489970 ) ) ;
#21877=CARTESIAN_POINT ( 'NONE',  ( 3.469446951953614189E-15, 40.00000000000000000, 8.999999999999992895 ) ) ;
#21891=CARTESIAN_POINT ( 'NONE',  ( 3.756430356250002323, 29.71562499938548640, 11.16877607737301226 ) ) ;
#21892=CARTESIAN_POINT ( 'NONE',  ( 1.071796769724494558, 28.18615380933863435, 4.999999999999992895 ) ) ;
#21898=CARTESIAN_POINT ( 'NONE',  ( 1.878215178125000939, 27.76562499938548356, 12.25316411605952283 ) ) ;
#21911=CARTESIAN_POINT ( 'NONE',  ( -1.878215178124998497, 29.04062499938548569, 12.25316411605951927 ) ) ;
#21916=CARTESIAN_POINT ( 'NONE',  ( -3.999999999999996447, 26.51874999877097139, 8.999999999999992895 ) ) ;
#21920=CARTESIAN_POINT ( 'NONE',  ( 3.756430356250002323, 27.91562499938548569, 11.16877607737301403 ) ) ;
#21945=CARTESIAN_POINT ( 'NONE',  ( -1.878215178124995832, 28.10312499938548569, 5.746835883940462963 ) ) ;
#21951=CARTESIAN_POINT ( 'NONE',  ( 3.756430356250003655, 29.64062499938548356, 8.999999999999992895 ) ) ;
#21960=CARTESIAN_POINT ( 'NONE',  ( 3.469446951953614189E-15, 40.00000000000000000, 8.999999999999992895 ) ) ;
#21972=CARTESIAN_POINT ( 'NONE',  ( -3.756430356249996105, 27.12812499938548427, 6.831223922626973533 ) ) ;
#21982=CARTESIAN_POINT ( 'NONE',  ( 4.000000000000003553, 28.60000000000000142, 8.999999999999992895 ) ) ;
#21998=EDGE_CURVE ( 'NONE', #24266, #9446, #22653, .T. ) ;
#21999=DIRECTION ( 'NONE',  ( 0.000000000000000000, 1.000000000000000000, 0.000000000000000000 ) ) ;
#22002=CARTESIAN_POINT ( 'NONE',  ( 4.000000000000001776, 29.01249999999999929, 11.30940107675849760 ) ) ;
#22019=CARTESIAN_POINT ( 'NONE',  ( 3.756430356250004099, 27.87812499938548427, 6.831223922626973533 ) ) ;
#22026=EDGE_CURVE ( 'NONE', #1168, #12794, #18596, .T. ) ;
#22036=CARTESIAN_POINT ( 'NONE',  ( -3.999999999999997335, 27.45624999877096784, 11.30940107675849404 ) ) ;
#22040=CARTESIAN_POINT ( 'NONE',  ( -3.756430356249997438, 27.31562499938548427, 11.16877607737301048 ) ) ;
#22051=CARTESIAN_POINT ( 'NONE',  ( -3.999999999999997335, 27.45624999877096784, 11.30940107675849404 ) ) ;
#22057=CARTESIAN_POINT ( 'NONE',  ( 2.000000000000000888, 25.37500000000000000, 12.46410161513774817 ) ) ;
#22063=CARTESIAN_POINT ( 'NONE',  ( 2.672651547586948120E-15, 29.64062499938548356, 13.33755215474602984 ) ) ;
#22082=CARTESIAN_POINT ( 'NONE',  ( -1.999999999999995781, 26.44374999877096855, 5.535898384862237620 ) ) ;
#22090=CARTESIAN_POINT ( 'NONE',  ( -1.878215178124995832, 26.64062499938548711, 5.746835883940462963 ) ) ;
#22108=VERTEX_POINT ( 'NONE', #803 ) ;
#22115=CARTESIAN_POINT ( 'NONE',  ( -1.999999999999998224, 29.35000000000000142, 12.46410161513774639 ) ) ;
#22125=( LENGTH_UNIT ( ) NAMED_UNIT ( * ) SI_UNIT ( .MILLI., .METRE. ) );
#22140=EDGE_CURVE ( 'NONE', #21434, #10206, #3570, .T. ) ;
#22149=VERTEX_POINT ( 'NONE', #9126 ) ;
#22151=CARTESIAN_POINT ( 'NONE',  ( 2.672651547586948120E-15, 27.72812499938548569, 13.33755215474602984 ) ) ;
#22170=EDGE_CURVE ( 'NONE', #18613, #22942, #8934, .T. ) ;
#22174=CARTESIAN_POINT ( 'NONE',  ( 4.000000000000003553, 27.23124999877096997, 6.690598923241489970 ) ) ;
#22179=CARTESIAN_POINT ( 'NONE',  ( -1.878215178124995832, 29.00312499938548427, 5.746835883940462963 ) ) ;
#22196=FACE_OUTER_BOUND ( 'NONE', #12561, .T. ) ;
#22204=CARTESIAN_POINT ( 'NONE',  ( 2.672651547586948120E-15, 25.92812499938548498, 13.33755215474602984 ) ) ;
#22218=EDGE_LOOP ( 'NONE', ( #11655, #16591, #4302, #12705 ) ) ;
#22232=CARTESIAN_POINT ( 'NONE',  ( 2.672651547586948120E-15, 25.47812499938548569, 13.33755215474603162 ) ) ;
#22287=CARTESIAN_POINT ( 'NONE',  ( 3.756430356250003655, 28.29062499938548569, 8.999999999999992895 ) ) ;
#22303=CARTESIAN_POINT ( 'NONE',  ( -1.999999999999998224, 27.94374999877096855, 12.46410161513774639 ) ) ;
#22308=CARTESIAN_POINT ( 'NONE',  ( -3.999999999999997335, 28.80624999877096926, 11.30940107675849404 ) ) ;
#22310=CARTESIAN_POINT ( 'NONE',  ( -1.999999999999998224, 27.94374999877096855, 12.46410161513774639 ) ) ;
#22323=CARTESIAN_POINT ( 'NONE',  ( 4.000000000000003553, 25.48750000000000071, 6.690598923241489970 ) ) ;
#22329=CARTESIAN_POINT ( 'NONE',  ( -3.756430356249995661, 25.77812499938548640, 6.831223922626973533 ) ) ;
#22346=ADVANCED_FACE ( 'NONE', ( #12643 ), #20475, .T. ) ;
#22353=CARTESIAN_POINT ( 'NONE',  ( 3.756430356250003211, 26.07812499938548356, 6.831223922626973533 ) ) ;
#22375=CARTESIAN_POINT ( 'NONE',  ( 2.000000000000003997, 28.67500000000000426, 5.535898384862238508 ) ) ;
#22379=PRODUCT ( 'dust cap', 'dust cap', '', ( #3337 ) ) ;
#22407=CARTESIAN_POINT ( 'NONE',  ( 3.756430356250002323, 26.45312499938548356, 11.16877607737301226 ) ) ;
#22423=CARTESIAN_POINT ( 'NONE',  ( 3.756430356250002323, 26.11562499938548498, 11.16877607737301226 ) ) ;
#22433=CARTESIAN_POINT ( 'NONE',  ( -1.071796769724487230, 25.52634618820330559, 4.999999999999992006 ) ) ;
#22452=CARTESIAN_POINT ( 'NONE',  ( 3.756430356250002323, 26.45312499938548356, 11.16877607737301226 ) ) ;
#22454=ORIENTED_EDGE ( 'NONE', *, *, #5202, .T. ) ;
#22482=CARTESIAN_POINT ( 'NONE',  ( -3.756430356249997438, 25.85312499938548569, 11.16877607737301048 ) ) ;
#22510=ADVANCED_BREP_SHAPE_REPRESENTATION ( '', ( #22659, #21036 ), #8945 ) ;
#22538=CARTESIAN_POINT ( 'NONE',  ( -3.999999999999997335, 29.25624999877096855, 11.30940107675849404 ) ) ;
#22543=CARTESIAN_POINT ( 'NONE',  ( 2.672651547586948120E-15, 29.52812499938548285, 13.33755215474602984 ) ) ;
#22564=CARTESIAN_POINT ( 'NONE',  ( -3.999999999999996447, 29.21874999877096712, 8.999999999999992895 ) ) ;
#22570=LINE ( 'NONE', #8313, #11232 ) ;
#22586=CARTESIAN_POINT ( 'NONE',  ( 3.469446951953614189E-15, 40.00000000000000000, 8.999999999999992895 ) ) ;
#22594=CARTESIAN_POINT ( 'NONE',  ( 3.735045420075836212E-15, 28.96562499938548640, 4.662447845253954171 ) ) ;
#22598=PLANE ( 'NONE',  #2057 ) ;
#22626=CARTESIAN_POINT ( 'NONE',  ( -3.756430356249996105, 28.92812499938548498, 6.831223922626973533 ) ) ;
#22640=VERTEX_POINT ( 'NONE', #1994 ) ;
#22653=LINE ( 'NONE', #6824, #6679 ) ;
#22659=MANIFOLD_SOLID_BREP ( 'Cavity1', #24656 ) ;
#22676=CARTESIAN_POINT ( 'NONE',  ( 3.369928719974892281E-15, 25.11250000000000426, 4.999999999999992006 ) ) ;
#22683=CARTESIAN_POINT ( 'NONE',  ( 2.620986760973688460E-15, 25.78750000000000142, 13.61880215351699874 ) ) ;
#22702=CARTESIAN_POINT ( 'NONE',  ( -1.878215178124998497, 26.45312499938548711, 12.25316411605951927 ) ) ;
#22707=CARTESIAN_POINT ( 'NONE',  ( -1.071796769724488563, 28.86115380933863506, 12.99999999999999289 ) ) ;
#22728=CARTESIAN_POINT ( 'NONE',  ( 2.672651547586948120E-15, 27.72812499938548569, 13.33755215474602984 ) ) ;
#22733=ORIENTED_EDGE ( 'NONE', *, *, #8784, .F. ) ;
#22738=ORIENTED_EDGE ( 'NONE', *, *, #6345, .F. ) ;
#22755=CARTESIAN_POINT ( 'NONE',  ( -3.756430356249997438, 27.65312499938548640, 11.16877607737301048 ) ) ;
#22770=EDGE_LOOP ( 'NONE', ( #11794, #2755, #12419, #9114 ) ) ;
#22806=CARTESIAN_POINT ( 'NONE',  ( -1.878215178124995832, 28.89062499938548356, 5.746835883940462963 ) ) ;
#22808=CARTESIAN_POINT ( 'NONE',  ( -3.999999999999996447, 28.31874999877096855, 8.999999999999992895 ) ) ;
#22809=CARTESIAN_POINT ( 'NONE',  ( 3.469446951953614189E-15, 34.00000000000000000, 8.999999999999992895 ) ) ;
#22815=CARTESIAN_POINT ( 'NONE',  ( -3.999999999999997335, 26.16250000000000142, 11.30940107675849404 ) ) ;
#22822=CARTESIAN_POINT ( 'NONE',  ( 3.752267015613588906E-15, 29.55624999877096926, 4.381197846482986158 ) ) ;
#22828=CARTESIAN_POINT ( 'NONE',  ( -1.071796769724487230, 28.67634618820330417, 4.999999999999992006 ) ) ;
#22835=DIRECTION ( 'NONE',  ( -0.000000000000000000, -1.000000000000000000, -0.000000000000000000 ) ) ;
#22850=CARTESIAN_POINT ( 'NONE',  ( 3.756430356250004099, 28.77812499938548285, 6.831223922626973533 ) ) ;
#22854=ORIENTED_EDGE ( 'NONE', *, *, #1964, .T. ) ;
#22874=CARTESIAN_POINT ( 'NONE',  ( -1.878215178124998497, 28.59062499938548285, 12.25316411605951927 ) ) ;
#22880=CARTESIAN_POINT ( 'NONE',  ( -1.878215178124995832, 25.40312499938548640, 5.746835883940462963 ) ) ;
#22881=FACE_OUTER_BOUND ( 'NONE', #24724, .T. ) ;
#22883=LINE ( 'NONE', #15296, #13911 ) ;
#22928=CARTESIAN_POINT ( 'NONE',  ( 3.756430356250002323, 29.60312499938548569, 11.16877607737301226 ) ) ;
#22942=VERTEX_POINT ( 'NONE', #9689 ) ;
#22949=CARTESIAN_POINT ( 'NONE',  ( -3.999999999999996003, 29.63124999877096499, 6.690598923241487306 ) ) ;
#22979=CARTESIAN_POINT ( 'NONE',  ( -3.756430356249996994, 28.96562499938548285, 8.999999999999992895 ) ) ;
#22991=CARTESIAN_POINT ( 'NONE',  ( -3.756430356249997438, 26.86562499938548498, 11.16877607737301048 ) ) ;
#23009=UNCERTAINTY_MEASURE_WITH_UNIT (LENGTH_MEASURE( 1.000000000000000082E-05 ), #22125, 'distance_accuracy_value', 'NONE');
#23017=CARTESIAN_POINT ( 'NONE',  ( -1.878215178124998497, 26.00312499938548783, 12.25316411605951927 ) ) ;
#23052=ORIENTED_EDGE ( 'NONE', *, *, #16833, .F. ) ;
#23054=EDGE_CURVE ( 'NONE', #7170, #16822, #7976, .T. ) ;
#23068=CARTESIAN_POINT ( 'NONE',  ( 3.752267015613588906E-15, 25.56250000000000000, 4.381197846482986158 ) ) ;
#23085=CARTESIAN_POINT ( 'NONE',  ( -1.999999999999998224, 27.10000000000000142, 12.46410161513774639 ) ) ;
#23086=CARTESIAN_POINT ( 'NONE',  ( 1.878215178125004048, 27.57812499938548711, 5.746835883940462963 ) ) ;
#23112=CARTESIAN_POINT ( 'NONE',  ( -1.878215178124998497, 28.14062499938548356, 12.25316411605951927 ) ) ;
#23117=CARTESIAN_POINT ( 'NONE',  ( -1.999999999999995781, 26.44374999877096855, 5.535898384862237620 ) ) ;
#23122=CARTESIAN_POINT ( 'NONE',  ( 1.878215178125000939, 25.62812499938548783, 12.25316411605952283 ) ) ;
#23134=CARTESIAN_POINT ( 'NONE',  ( 4.000000000000001776, 28.95624999877097494, 11.30940107675849760 ) ) ;
#23136=( BOUNDED_CURVE ( )  B_SPLINE_CURVE ( 2, ( #23175, #25384, #11013, #13504, #11523, #7471, #3548, #5256, #9317 ),
 .UNSPECIFIED., .F., .F. ) 
 B_SPLINE_CURVE_WITH_KNOTS ( ( 3, 2, 2, 2, 3 ),
 ( 0.1250000000000000000, 0.1333333333333333315, 0.1499999999999999944, 0.1666666666666666574, 0.1749999999999999889 ),
 .UNSPECIFIED. ) 
 CURVE ( )  GEOMETRIC_REPRESENTATION_ITEM ( )  RATIONAL_B_SPLINE_CURVE ( ( 0.9330127018922194093, 0.9330127018922194093, 1.000000000000000000, 0.8660254037844387076, 1.000000000000000000, 0.8660254037844387076, 1.000000000000000000, 0.9330127018922194093, 0.9330127018922194093 ) ) 
 REPRESENTATION_ITEM ( '' )  );
#23139=CARTESIAN_POINT ( 'NONE',  ( -3.756430356249996105, 27.57812499938548356, 6.831223922626973533 ) ) ;
#23157=ADVANCED_FACE ( 'NONE', ( #19865 ), #6017, .F. ) ;
#23159=CARTESIAN_POINT ( 'NONE',  ( -1.999999999999995781, 29.14374999877096784, 5.535898384862237620 ) ) ;
#23170=CARTESIAN_POINT ( 'NONE',  ( 3.469446951953614189E-15, 40.00000000000000000, 4.999999999999992006 ) ) ;
#23175=CARTESIAN_POINT ( 'NONE',  ( 3.834746474454188013E-15, 25.56250000000000000, 4.999999999999992006 ) ) ;
#23183=CARTESIAN_POINT ( 'NONE',  ( 1.859271017917182139E-15, 26.68750000000000000, 12.99999999999999289 ) ) ;
#23185=CARTESIAN_POINT ( 'NONE',  ( -3.999999999999997335, 27.51250000000000284, 11.30940107675849404 ) ) ;
#23189=CARTESIAN_POINT ( 'NONE',  ( 3.469446951953614189E-15, 40.00000000000000000, 4.999999999999992006 ) ) ;
#23203=CARTESIAN_POINT ( 'NONE',  ( 3.756430356250003655, 27.95312499938548711, 8.999999999999992895 ) ) ;
#23229=CARTESIAN_POINT ( 'NONE',  ( -1.878215178124995832, 28.44062499938548427, 5.746835883940462963 ) ) ;
#23239=CARTESIAN_POINT ( 'NONE',  ( 3.756430356250003211, 25.74062499938548498, 6.831223922626973533 ) ) ;
#23267=DIRECTION ( 'NONE',  ( -0.000000000000000000, -1.000000000000000000, -0.000000000000000000 ) ) ;
#23307=CARTESIAN_POINT ( 'NONE',  ( 4.000000000000003553, 28.18750000000000000, 6.690598923241489970 ) ) ;
#23327=CARTESIAN_POINT ( 'NONE',  ( 2.672651547586948120E-15, 28.74062499938548498, 13.33755215474602984 ) ) ;
#23352=CARTESIAN_POINT ( 'NONE',  ( -3.756430356249995661, 29.37812499938548427, 6.831223922626973533 ) ) ;
#23364=DIRECTION ( 'NONE',  ( -0.000000000000000000, -1.000000000000000000, -0.000000000000000000 ) ) ;
#23383=DIRECTION ( 'NONE',  ( -0.8660254037844397068, -0.4999999999999983347, 0.000000000000000000 ) ) ;
#23386=CARTESIAN_POINT ( 'NONE',  ( 3.834746474454188013E-15, 25.95624999877096428, 4.999999999999992006 ) ) ;
#23389=EDGE_LOOP ( 'NONE', ( #221, #6295, #5964, #1531 ) ) ;
#23392=CARTESIAN_POINT ( 'NONE',  ( 2.672651547586948120E-15, 28.29062499938548569, 13.33755215474602984 ) ) ;
#23408=CARTESIAN_POINT ( 'NONE',  ( -1.071796769724488563, 29.31115380933863790, 12.99999999999999289 ) ) ;
#23442=CARTESIAN_POINT ( 'NONE',  ( -3.999999999999997335, 28.41249999999999787, 11.30940107675849404 ) ) ;
#23461=VECTOR ( 'NONE', #24747, 1000.000000000000000 ) ;
#23464=CARTESIAN_POINT ( 'NONE',  ( -3.756430356249996994, 28.62812499938548427, 8.999999999999992895 ) ) ;
#23473=CARTESIAN_POINT ( 'NONE',  ( -1.878215178124998497, 25.89062499938548356, 12.25316411605951927 ) ) ;
#23480=AXIS2_PLACEMENT_3D ( 'NONE', #13618, #14004, #10067 ) ;
#23491=CARTESIAN_POINT ( 'NONE',  ( -1.878215178124995832, 29.34062499938548285, 5.746835883940462963 ) ) ;
#23495=CARTESIAN_POINT ( 'NONE',  ( -1.999999999999998224, 25.69374999877097210, 12.46410161513774639 ) ) ;
#23499=CARTESIAN_POINT ( 'NONE',  ( -3.756430356249996994, 25.92812499938548498, 8.999999999999992895 ) ) ;
#23525=CARTESIAN_POINT ( 'NONE',  ( 3.756430356250004099, 27.54062499938548569, 6.831223922626973533 ) ) ;
#23539=ORIENTED_EDGE ( 'NONE', *, *, #7122, .F. ) ;
#23543=EDGE_CURVE ( 'NONE', #3732, #12422, #19833, .T. ) ;
#23562=CARTESIAN_POINT ( 'NONE',  ( 3.469446951953614189E-15, 40.00000000000000000, 8.999999999999992895 ) ) ;
#23576=CARTESIAN_POINT ( 'NONE',  ( 3.752267015613588906E-15, 26.46250000000000213, 4.381197846482986158 ) ) ;
#23594=CARTESIAN_POINT ( 'NONE',  ( -3.756430356249997882, 26.86562499938548498, 11.16877607737301226 ) ) ;
#23602=CARTESIAN_POINT ( 'NONE',  ( 3.756430356250003655, 25.14062499938548356, 8.999999999999992895 ) ) ;
#23615=CARTESIAN_POINT ( 'NONE',  ( 2.000000000000000888, 29.36874999877096926, 12.46410161513774817 ) ) ;
#23620=VERTEX_POINT ( 'NONE', #16177 ) ;
#23621=CARTESIAN_POINT ( 'NONE',  ( 2.000000000000000888, 26.66874999877096641, 12.46410161513774817 ) ) ;
#23625=CARTESIAN_POINT ( 'NONE',  ( 1.878215178125000939, 27.87812499938548427, 12.25316411605952283 ) ) ;
#23634=ADVANCED_FACE ( 'NONE', ( #22196 ), #3758, .T. ) ;
#23648=CARTESIAN_POINT ( 'NONE',  ( 3.756430356250002323, 28.81562499938548427, 11.16877607737301226 ) ) ;
#23658=ORIENTED_EDGE ( 'NONE', *, *, #2345, .F. ) ;
#23679=DIRECTION ( 'NONE',  ( 0.000000000000000000, 0.000000000000000000, -1.000000000000000000 ) ) ;
#23681=CARTESIAN_POINT ( 'NONE',  ( 2.000000000000003997, 28.67500000000000426, 5.535898384862238508 ) ) ;
#23692=CARTESIAN_POINT ( 'NONE',  ( -3.999999999999996447, 27.47499999999999787, 8.999999999999992895 ) ) ;
#23701=CARTESIAN_POINT ( 'NONE',  ( -3.999999999999996447, 29.27500000000000213, 8.999999999999992895 ) ) ;
#23717=CARTESIAN_POINT ( 'NONE',  ( 3.756430356250002323, 25.55312499938548143, 11.16877607737301226 ) ) ;
#23733=CARTESIAN_POINT ( 'NONE',  ( 3.756430356250003655, 29.19062499938548072, 8.999999999999992895 ) ) ;
#23734=VECTOR ( 'NONE', #9707, 1000.000000000000000 ) ;
#23740=CARTESIAN_POINT ( 'NONE',  ( -3.999999999999997335, 27.90624999877097068, 11.30940107675849404 ) ) ;
#23744=CARTESIAN_POINT ( 'NONE',  ( -3.756430356249996105, 28.59062499938548640, 6.831223922626973533 ) ) ;
#23764=CARTESIAN_POINT ( 'NONE',  ( 2.000000000000003997, 25.52500000000000213, 5.535898384862238508 ) ) ;
#23769=CARTESIAN_POINT ( 'NONE',  ( 1.626862140677534194E-14, 28.03750000000000497, 12.99999999999999289 ) ) ;
#23770=CARTESIAN_POINT ( 'NONE',  ( -1.878215178124995832, 27.65312499938548640, 5.746835883940462963 ) ) ;
#23776=CARTESIAN_POINT ( 'NONE',  ( 4.000000000000001776, 27.21250000000000213, 11.30940107675849760 ) ) ;
#23779=ORIENTED_EDGE ( 'NONE', *, *, #20242, .T. ) ;
#23814=( BOUNDED_CURVE ( )  B_SPLINE_CURVE ( 2, ( #6373, #24288, #22057, #8207, #8084, #22323, #23764, #2062, #10279 ),
 .UNSPECIFIED., .F., .F. ) 
 B_SPLINE_CURVE_WITH_KNOTS ( ( 3, 2, 2, 2, 3 ),
 ( 0.07500000000000001110, 0.08333333333333332871, 0.1000000000000000056, 0.1166666666666666685, 0.1250000000000000000 ),
 .UNSPECIFIED. ) 
 CURVE ( )  GEOMETRIC_REPRESENTATION_ITEM ( )  RATIONAL_B_SPLINE_CURVE ( ( 0.9330127018922192983, 0.9330127018922194093, 1.000000000000000000, 0.8660254037844387076, 1.000000000000000000, 0.8660254037844387076, 1.000000000000000000, 0.9330127018922194093, 0.9330127018922194093 ) ) 
 REPRESENTATION_ITEM ( '' )  );
#23815=AXIS2_PLACEMENT_3D ( 'NONE', #6895, #7016, #14878 ) ;
#23824=VERTEX_POINT ( 'NONE', #18785 ) ;
#23869=CARTESIAN_POINT ( 'NONE',  ( 3.834746474454188013E-15, 27.36250000000000426, 4.999999999999992006 ) ) ;
#23876=CARTESIAN_POINT ( 'NONE',  ( 1.626862140677534194E-14, 28.03750000000000497, 12.99999999999999289 ) ) ;
#23880=CARTESIAN_POINT ( 'NONE',  ( 3.752267015613588906E-15, 26.85624999877096641, 4.381197846482986158 ) ) ;
#23883=CARTESIAN_POINT ( 'NONE',  ( 3.469446951953614189E-15, 34.00000000000000000, 8.999999999999992895 ) ) ;
#23885=CARTESIAN_POINT ( 'NONE',  ( 3.756430356250002323, 28.81562499938548427, 11.16877607737301403 ) ) ;
#23891=ORIENTED_EDGE ( 'NONE', *, *, #9608, .T. ) ;
#23902=VECTOR ( 'NONE', #14923, 1000.000000000000000 ) ;
#23911=CARTESIAN_POINT ( 'NONE',  ( 1.878215178125004048, 27.57812499938548711, 5.746835883940462963 ) ) ;
#23918=CYLINDRICAL_SURFACE ( 'NONE', #17546, 4.000000000000000000 ) ;
#23937=CARTESIAN_POINT ( 'NONE',  ( 3.756430356250003655, 26.04062499938548569, 8.999999999999992895 ) ) ;
#23948=CARTESIAN_POINT ( 'NONE',  ( 2.000000000000000888, 28.52500000000000213, 12.46410161513774817 ) ) ;
#23961=CARTESIAN_POINT ( 'NONE',  ( 2.620986760973688460E-15, 28.48750000000000071, 13.61880215351699874 ) ) ;
#23972=CARTESIAN_POINT ( 'NONE',  ( -1.999999999999995781, 29.19999999999999929, 5.535898384862237620 ) ) ;
#23987=CARTESIAN_POINT ( 'NONE',  ( 1.878215178125000939, 25.96562499938548285, 12.25316411605952283 ) ) ;
#23996=CARTESIAN_POINT ( 'NONE',  ( -3.999999999999996447, 27.47499999999999787, 8.999999999999992895 ) ) ;
#24000=CARTESIAN_POINT ( 'NONE',  ( 3.959305671612554781E-15, 40.00000000000000000, 12.99999999999999289 ) ) ;
#24005=CARTESIAN_POINT ( 'NONE',  ( -3.999999999999996447, 26.96874999877096712, 8.999999999999992895 ) ) ;
#24010=CARTESIAN_POINT ( 'NONE',  ( 1.878215178125000939, 29.22812499938548569, 12.25316411605952283 ) ) ;
#24018=ADVANCED_FACE ( 'NONE', ( #1395 ), #9096, .T. ) ;
#24030=ORIENTED_EDGE ( 'NONE', *, *, #841, .T. ) ;
#24033=CARTESIAN_POINT ( 'NONE',  ( -3.756430356249997882, 25.40312499938548285, 11.16877607737301226 ) ) ;
#24035=DIRECTION ( 'NONE',  ( 0.000000000000000000, 1.000000000000000000, 0.000000000000000000 ) ) ;
#24058=CARTESIAN_POINT ( 'NONE',  ( 3.735045420075836212E-15, 27.05312499938548498, 4.662447845253954171 ) ) ;
#24076=ORIENTED_EDGE ( 'NONE', *, *, #25395, .T. ) ;
#24101=CARTESIAN_POINT ( 'NONE',  ( 3.756430356250003655, 29.30312499938548498, 8.999999999999992895 ) ) ;
#24108=CARTESIAN_POINT ( 'NONE',  ( -3.756430356249995661, 28.02812499938548640, 6.831223922626973533 ) ) ;
#24116=EDGE_CURVE ( 'NONE', #1665, #15816, #1750, .T. ) ;
#24121=CARTESIAN_POINT ( 'NONE',  ( 5.577813053751546416E-15, 25.33750000000000213, 12.99999999999999289 ) ) ;
#24125=CARTESIAN_POINT ( 'NONE',  ( -3.999999999999997335, 28.80624999877096926, 11.30940107675849404 ) ) ;
#24129=CARTESIAN_POINT ( 'NONE',  ( -1.878215178124998497, 28.70312499938548356, 12.25316411605951927 ) ) ;
#24153=CARTESIAN_POINT ( 'NONE',  ( -1.878215178124995832, 25.29062499938548569, 5.746835883940462963 ) ) ;
#24173=CARTESIAN_POINT ( 'NONE',  ( -3.999999999999996447, 26.96874999877096712, 8.999999999999992895 ) ) ;
#24176=CARTESIAN_POINT ( 'NONE',  ( -3.999999999999997335, 26.55624999877096570, 11.30940107675849404 ) ) ;
#24185=CARTESIAN_POINT ( 'NONE',  ( -3.756430356249997438, 27.20312499938548356, 11.16877607737301048 ) ) ;
#24238=EDGE_CURVE ( 'NONE', #8387, #9446, #4667, .T. ) ;
#24241=CARTESIAN_POINT ( 'NONE',  ( 4.000000000000001776, 28.50624999877096855, 11.30940107675849760 ) ) ;
#24242=CARTESIAN_POINT ( 'NONE',  ( -3.756430356249996994, 26.71562499938548285, 8.999999999999992895 ) ) ;
#24261=CARTESIAN_POINT ( 'NONE',  ( 4.000000000000003553, 26.78124999877097068, 6.690598923241489970 ) ) ;
#24266=VERTEX_POINT ( 'NONE', #597 ) ;
#24270=CARTESIAN_POINT ( 'NONE',  ( -3.999999999999997335, 25.65624999877097068, 11.30940107675849404 ) ) ;
#24285=AXIS2_PLACEMENT_3D ( 'NONE', #17502, #13201, #13468 ) ;
#24288=CARTESIAN_POINT ( 'NONE',  ( 1.071796769724494336, 25.35759618943234628, 12.99999999999999467 ) ) ;
#24294=CARTESIAN_POINT ( 'NONE',  ( -3.756430356249996994, 25.81562499938548427, 8.999999999999992895 ) ) ;
#24315=EDGE_CURVE ( 'NONE', #22640, #14520, #7084, .T. ) ;
#24325=CARTESIAN_POINT ( 'NONE',  ( 1.878215178125004048, 27.46562499938548640, 5.746835883940462963 ) ) ;
#24332=CARTESIAN_POINT ( 'NONE',  ( -3.999999999999996447, 27.92500000000000071, 8.999999999999992895 ) ) ;
#24348=CARTESIAN_POINT ( 'NONE',  ( 4.000000000000003553, 29.05000000000000071, 8.999999999999992895 ) ) ;
#24359=( NAMED_UNIT ( * ) SI_UNIT ( $, .STERADIAN. ) SOLID_ANGLE_UNIT ( ) );
#24367=CARTESIAN_POINT ( 'NONE',  ( 3.834746474454188013E-15, 26.01249999999999574, 4.999999999999992006 ) ) ;
#24382=CARTESIAN_POINT ( 'NONE',  ( 4.000000000000003553, 28.58124999877096784, 6.690598923241489970 ) ) ;
#24383=CARTESIAN_POINT ( 'NONE',  ( -3.756430356249997882, 26.30312499938548498, 11.16877607737301226 ) ) ;
#24388=EDGE_CURVE ( 'NONE', #23620, #22640, #17628, .T. ) ;
#24399=CARTESIAN_POINT ( 'NONE',  ( 3.756430356250004099, 25.74062499938548143, 6.831223922626973533 ) ) ;
#24407=DIRECTION ( 'NONE',  ( -0.000000000000000000, -1.000000000000000000, -0.000000000000000000 ) ) ;
#24423=CARTESIAN_POINT ( 'NONE',  ( 3.756430356250003655, 26.04062499938548569, 8.999999999999992895 ) ) ;
#24450=CARTESIAN_POINT ( 'NONE',  ( 1.878215178125004048, 25.66562499938548569, 5.746835883940462963 ) ) ;
#24470=CARTESIAN_POINT ( 'NONE',  ( 3.756430356250003655, 25.14062499938548356, 8.999999999999992895 ) ) ;
#24501=CARTESIAN_POINT ( 'NONE',  ( -3.756430356249996994, 28.96562499938548285, 8.999999999999992895 ) ) ;
#24502=DIRECTION ( 'NONE',  ( 0.000000000000000000, 0.000000000000000000, 1.000000000000000000 ) ) ;
#24514=CARTESIAN_POINT ( 'NONE',  ( -1.878215178124995832, 26.30312499938548498, 5.746835883940462963 ) ) ;
#24520=CARTESIAN_POINT ( 'NONE',  ( 2.000000000000003997, 26.36874999877096926, 5.535898384862238508 ) ) ;
#24538=CARTESIAN_POINT ( 'NONE',  ( -1.878215178124995832, 25.74062499938548498, 5.746835883940462963 ) ) ;
#24567=CARTESIAN_POINT ( 'NONE',  ( 3.756430356250003211, 29.22812499938548569, 6.831223922626973533 ) ) ;
#24624=CARTESIAN_POINT ( 'NONE',  ( 3.735045420075836212E-15, 29.30312499938548498, 4.662447845253954171 ) ) ;
#24627=CYLINDRICAL_SURFACE ( 'NONE', #18853, 4.000000000000000000 ) ;
#24645=CARTESIAN_POINT ( 'NONE',  ( -1.878215178124998497, 25.55312499938548854, 12.25316411605951927 ) ) ;
#24656=CLOSED_SHELL ( 'NONE', ( #2399, #17222, #9644, #7705, #24018, #5726, #13559, #21700, #9631, #16205, #2896, #24674, #12986, #23634, #270, #17544, #8535, #1958, #6101, #2845, #1005, #6271, #22346, #11633, #25516, #19665, #17807, #23157, #16136, #1326, #1874, #12057 ) ) ;
#24666=DIRECTION ( 'NONE',  ( 0.000000000000000000, 0.000000000000000000, -1.000000000000000000 ) ) ;
#24674=ADVANCED_FACE ( 'NONE', ( #7186 ), #15174, .T. ) ;
#24676=CARTESIAN_POINT ( 'NONE',  ( 1.626862140677534194E-14, 27.58750000000000213, 12.99999999999999289 ) ) ;
#24678=CARTESIAN_POINT ( 'NONE',  ( 2.672651547586948120E-15, 27.27812499938548285, 13.33755215474602984 ) ) ;
#24683=CARTESIAN_POINT ( 'NONE',  ( 3.469446951953614189E-15, 46.00000000000000000, 8.999999999999992895 ) ) ;
#24708=CARTESIAN_POINT ( 'NONE',  ( 3.735045420075836212E-15, 28.40312499938548640, 4.662447845253954171 ) ) ;
#24724=EDGE_LOOP ( 'NONE', ( #8087, #19975, #6965, #19502 ) ) ;
#24727=ORIENTED_EDGE ( 'NONE', *, *, #300, .T. ) ;
#24747=DIRECTION ( 'NONE',  ( -0.000000000000000000, -1.000000000000000000, -0.000000000000000000 ) ) ;
#24768=CARTESIAN_POINT ( 'NONE',  ( 3.752267015613588906E-15, 26.01249999999999929, 4.381197846482986158 ) ) ;
#24769=CARTESIAN_POINT ( 'NONE',  ( -3.999999999999997335, 28.35624999877096997, 11.30940107675849404 ) ) ;
#24785=CARTESIAN_POINT ( 'NONE',  ( -3.756430356249997882, 26.41562499938548569, 11.16877607737301226 ) ) ;
#24792=ORIENTED_EDGE ( 'NONE', *, *, #25472, .T. ) ;
#24797=CARTESIAN_POINT ( 'NONE',  ( 3.469446951953614189E-15, 40.00000000000000000, 8.999999999999992895 ) ) ;
#24801=APPLICATION_CONTEXT ( 'automotive_design' ) ;
#24811=CARTESIAN_POINT ( 'NONE',  ( 4.000000000000003553, 27.70000000000000284, 8.999999999999992895 ) ) ;
#24814=CARTESIAN_POINT ( 'NONE',  ( -1.878215178124995832, 27.99062499938548143, 5.746835883940462963 ) ) ;
#24817=DIRECTION ( 'NONE',  ( 0.000000000000000000, -0.000000000000000000, 1.000000000000000000 ) ) ;
#24843=CARTESIAN_POINT ( 'NONE',  ( -1.878215178124998497, 27.69062499938548427, 12.25316411605951927 ) ) ;
#24849=CARTESIAN_POINT ( 'NONE',  ( 3.756430356250004099, 26.19062499938548783, 6.831223922626973533 ) ) ;
#24854=CARTESIAN_POINT ( 'NONE',  ( 3.469446951953614189E-15, 40.00000000000000000, 4.999999999999992006 ) ) ;
#24855=FACE_OUTER_BOUND ( 'NONE', #19880, .T. ) ;
#24895=CARTESIAN_POINT ( 'NONE',  ( 3.735045420075836212E-15, 28.85312499938548569, 4.662447845253954171 ) ) ;
#24897=EDGE_CURVE ( 'NONE', #15816, #22149, #25647, .T. ) ;
#24898=CARTESIAN_POINT ( 'NONE',  ( -3.137519842735244810E-15, 26.46249999999999858, 4.999999999999991118 ) ) ;
#24901=CARTESIAN_POINT ( 'NONE',  ( -1.999999999999995781, 28.30000000000000071, 5.535898384862237620 ) ) ;
#24911=CARTESIAN_POINT ( 'NONE',  ( 4.000000000000003553, 29.48124999877096997, 6.690598923241489970 ) ) ;
#24917=CARTESIAN_POINT ( 'NONE',  ( 4.000000000000003553, 26.29374999877096997, 8.999999999999992895 ) ) ;
#24934=CARTESIAN_POINT ( 'NONE',  ( -1.878215178124998497, 26.79062499938548214, 12.25316411605951927 ) ) ;
#24939=CARTESIAN_POINT ( 'NONE',  ( -1.057460391440397258E-14, 28.71250000000000213, 4.999999999999992006 ) ) ;
#24944=CARTESIAN_POINT ( 'NONE',  ( -3.756430356249996994, 26.82812499938548711, 8.999999999999992895 ) ) ;
#24952=( BOUNDED_CURVE ( )  B_SPLINE_CURVE ( 2, ( #7024, #25077, #21153, #11196, #21532, #7295, #11583, #11077, #19556, #11467, #23122, #19176, #11334, #23239, #19438, #5322, #17481, #19055, #23499, #1273, #5205, #17366, #1140, #13302, #9113, #1529, #13183, #25332, #3224, #1658, #9257, #17245, #15391, #17102, #7163, #3614, #25453, #25215, #5452, #16979, #15272, #21275, #24944, #22991, #3359, #19317, #1412, #13444, #9499, #21414, #7538, #15533, #5076, #13056, #25841, #22040, #19940, #8066, #20205, #218, #19821, #15912, #5703, #9635, #19698, #11968, #7924, #15659, #17613, #1797, #23625, #21920, #6215, #2043, #7674, #6090, #25714, #4002, #10011, #16048, #18006, #10141, #2180, #20078, #17869, #13682, #12238, #21796, #4124, #23744, #21655, #8188, #24129, #1922, #14075, #23885, #18145, #16166, #14206, #12102, #22179, #5969, #9766, #4264, #25591, #3738, #24010, #94, #11721, #17744, #15775, #7796, #5831, #13818, #3879, #11850, #9883, #13952, #4904, #8579, #728 ),
 .UNSPECIFIED., .F., .F. ) 
 B_SPLINE_CURVE_WITH_KNOTS ( ( 3, 2, 2, 2, 2, 2, 2, 2, 2, 2, 2, 2, 2, 2, 2, 2, 2, 2, 2, 2, 2, 2, 2, 2, 2, 2, 2, 2, 2, 2, 2, 2, 2, 2, 2, 2, 2, 2, 2, 2, 2, 2, 2, 2, 2, 2, 2, 2, 2, 2, 2, 2, 2, 2, 2, 2, 2, 2, 2, 2, 3 ),
 ( 0.000000000000000000, 0.01666666666666666644, 0.03333333333333333287, 0.05000000000000000278, 0.06666666666666666574, 0.08333333333333332871, 0.1000000000000000056, 0.1166666666666666685, 0.1333333333333333315, 0.1499999999999999944, 0.1666666666666666574, 0.1833333333333333204, 0.2000000000000000111, 0.2166666666666666741, 0.2333333333333333370, 0.2500000000000000000, 0.2666666666666666630, 0.2833333333333333259, 0.2999999999999999889, 0.3166666666666666519, 0.3333333333333333148, 0.3499999999999999778, 0.3666666666666666408, 0.3833333333333333592, 0.4000000000000000222, 0.4166666666666666852, 0.4333333333333333481, 0.4500000000000000111, 0.4666666666666666741, 0.4833333333333333370, 0.5000000000000000000, 0.5166666666666667185, 0.5333333333333333259, 0.5500000000000000444, 0.5666666666666666519, 0.5833333333333333703, 0.5999999999999999778, 0.6166666666666666963, 0.6333333333333333037, 0.6500000000000000222, 0.6666666666666666297, 0.6833333333333333481, 0.6999999999999999556, 0.7166666666666666741, 0.7333333333333332815, 0.7500000000000000000, 0.7666666666666667185, 0.7833333333333333259, 0.8000000000000000444, 0.8166666666666666519, 0.8333333333333333703, 0.8499999999999999778, 0.8666666666666666963, 0.8833333333333333037, 0.9000000000000000222, 0.9166666666666666297, 0.9333333333333333481, 0.9499999999999999556, 0.9666666666666666741, 0.9833333333333332815, 1.000000000000000000 ),
 .UNSPECIFIED. ) 
 CURVE ( )  GEOMETRIC_REPRESENTATION_ITEM ( )  RATIONAL_B_SPLINE_CURVE ( ( 1.000000000000000000, 0.8660254037844387076, 1.000000000000000000, 0.8660254037844387076, 1.000000000000000000, 0.8660254037844387076, 1.000000000000000000, 0.8660254037844387076, 1.000000000000000000, 0.8660254037844387076, 1.000000000000000000, 0.8660254037844387076, 1.000000000000000000, 0.8660254037844387076, 1.000000000000000000, 0.8660254037844387076, 1.000000000000000000, 0.8660254037844387076, 1.000000000000000000, 0.8660254037844387076, 1.000000000000000000, 0.8660254037844387076, 1.000000000000000000, 0.8660254037844387076, 1.000000000000000000, 0.8660254037844387076, 1.000000000000000000, 0.8660254037844387076, 1.000000000000000000, 0.8660254037844387076, 1.000000000000000000, 0.8660254037844387076, 1.000000000000000000, 0.8660254037844387076, 1.000000000000000000, 0.8660254037844387076, 1.000000000000000000, 0.8660254037844387076, 1.000000000000000000, 0.8660254037844387076, 1.000000000000000000, 0.8660254037844387076, 1.000000000000000000, 0.8660254037844387076, 1.000000000000000000, 0.8660254037844387076, 1.000000000000000000, 0.8660254037844387076, 1.000000000000000000, 0.8660254037844387076, 1.000000000000000000, 0.8660254037844387076, 1.000000000000000000, 0.8660254037844387076, 1.000000000000000000, 0.8660254037844387076, 1.000000000000000000, 0.8660254037844387076, 1.000000000000000000, 0.8660254037844387076, 1.000000000000000000, 0.8660254037844387076, 1.000000000000000000, 0.8660254037844387076, 1.000000000000000000, 0.8660254037844387076, 1.000000000000000000, 0.8660254037844387076, 1.000000000000000000, 0.8660254037844387076, 1.000000000000000000, 0.8660254037844387076, 1.000000000000000000, 0.8660254037844387076, 1.000000000000000000, 0.8660254037844387076, 1.000000000000000000, 0.8660254037844387076, 1.000000000000000000, 0.8660254037844387076, 1.000000000000000000, 0.8660254037844387076, 1.000000000000000000, 0.8660254037844387076, 1.000000000000000000, 0.8660254037844387076, 1.000000000000000000, 0.8660254037844387076, 1.000000000000000000, 0.8660254037844387076, 1.000000000000000000, 0.8660254037844387076, 1.000000000000000000, 0.8660254037844387076, 1.000000000000000000, 0.8660254037844387076, 1.000000000000000000, 0.8660254037844387076, 1.000000000000000000, 0.8660254037844387076, 1.000000000000000000, 0.8660254037844387076, 1.000000000000000000, 0.8660254037844387076, 1.000000000000000000, 0.8660254037844387076, 1.000000000000000000, 0.8660254037844387076, 1.000000000000000000, 0.8660254037844387076, 1.000000000000000000, 0.8660254037844387076, 1.000000000000000000, 0.8660254037844387076, 1.000000000000000000, 0.8660254037844387076, 1.000000000000000000, 0.8660254037844387076, 1.000000000000000000, 0.8660254037844387076, 1.000000000000000000 ) ) 
 REPRESENTATION_ITEM ( '' )  );
#24954=CARTESIAN_POINT ( 'NONE',  ( 2.000000000000003997, 29.06874999877096855, 5.535898384862238508 ) ) ;
#24961=CARTESIAN_POINT ( 'NONE',  ( -1.878215178124998497, 29.04062499938548569, 12.25316411605951927 ) ) ;
#24963=DIRECTION ( 'NONE',  ( 0.000000000000000000, 0.000000000000000000, 1.000000000000000000 ) ) ;
#24967=FACE_OUTER_BOUND ( 'NONE', #2987, .T. ) ;
#24971=VERTEX_POINT ( 'NONE', #12245 ) ;
#25016=CARTESIAN_POINT ( 'NONE',  ( 1.878215178125004048, 28.36562499938548143, 5.746835883940462963 ) ) ;
#25017=CARTESIAN_POINT ( 'NONE',  ( 1.071796769724492338, 27.10134618820329777, 12.99999999999999467 ) ) ;
#25037=CARTESIAN_POINT ( 'NONE',  ( 3.735045420075836212E-15, 27.16562499938548569, 4.662447845253954171 ) ) ;
#25043=CARTESIAN_POINT ( 'NONE',  ( 4.000000000000001776, 26.25624999877096855, 11.30940107675849760 ) ) ;
#25065=CARTESIAN_POINT ( 'NONE',  ( -3.756430356249997882, 27.20312499938548001, 11.16877607737301226 ) ) ;
#25072=CARTESIAN_POINT ( 'NONE',  ( 4.000000000000001776, 26.70624999877097139, 11.30940107675849760 ) ) ;
#25077=CARTESIAN_POINT ( 'NONE',  ( 3.756430356250003211, 25.29062499938548569, 6.831223922626973533 ) ) ;
#25094=CARTESIAN_POINT ( 'NONE',  ( -1.057460391440397258E-14, 29.10624999877096641, 4.999999999999992006 ) ) ;
#25096=CARTESIAN_POINT ( 'NONE',  ( -3.756430356249996105, 29.37812499938548427, 6.831223922626973533 ) ) ;
#25102=CARTESIAN_POINT ( 'NONE',  ( 1.878215178125000939, 26.07812499938548356, 12.25316411605952283 ) ) ;
#25103=CARTESIAN_POINT ( 'NONE',  ( 4.000000000000001776, 27.60624999877096641, 11.30940107675849760 ) ) ;
#25119=EDGE_CURVE ( 'NONE', #13240, #9674, #5182, .T. ) ;
#25157=CARTESIAN_POINT ( 'NONE',  ( 4.000000000000001776, 27.21250000000000213, 11.30940107675849760 ) ) ;
#25177=CARTESIAN_POINT ( 'NONE',  ( -1.878215178124998497, 26.90312499938548285, 12.25316411605951927 ) ) ;
#25189=CARTESIAN_POINT ( 'NONE',  ( 3.756430356250003655, 25.25312499938548427, 8.999999999999992895 ) ) ;
#25197=EDGE_CURVE ( 'NONE', #23824, #16937, #2193, .T. ) ;
#25206=CARTESIAN_POINT ( 'NONE',  ( 3.735045420075836212E-15, 27.95312499938548001, 4.662447845253954171 ) ) ;
#25215=CARTESIAN_POINT ( 'NONE',  ( 3.756430356250003211, 26.64062499938548356, 6.831223922626973533 ) ) ;
#25240=EDGE_LOOP ( 'NONE', ( #19120, #16379, #9589, #897 ) ) ;
#25246=ORIENTED_EDGE ( 'NONE', *, *, #16004, .T. ) ;
#25280=CARTESIAN_POINT ( 'NONE',  ( 4.000000000000001776, 28.11250000000000426, 11.30940107675849760 ) ) ;
#25299=CARTESIAN_POINT ( 'NONE',  ( -1.878215178124998497, 28.70312499938548356, 12.25316411605951927 ) ) ;
#25301=EDGE_CURVE ( 'NONE', #9674, #18613, #9598, .T. ) ;
#25302=ORIENTED_EDGE ( 'NONE', *, *, #3855, .T. ) ;
#25321=CARTESIAN_POINT ( 'NONE',  ( 4.000000000000001776, 28.11250000000000071, 11.30940107675849760 ) ) ;
#25332=CARTESIAN_POINT ( 'NONE',  ( 3.735045420075836212E-15, 26.26562499938548356, 4.662447845253954171 ) ) ;
#25350=CARTESIAN_POINT ( 'NONE',  ( 3.735045420075836212E-15, 25.81562499938548783, 4.662447845253954171 ) ) ;
#25351=CARTESIAN_POINT ( 'NONE',  ( -3.999999999999997335, 29.70624999877096784, 11.30940107675849404 ) ) ;
#25366=CARTESIAN_POINT ( 'NONE',  ( -1.071796769724493448, 29.12634618820329990, 4.999999999999995559 ) ) ;
#25384=CARTESIAN_POINT ( 'NONE',  ( -1.071796769724487230, 25.58259618943233704, 4.999999999999992006 ) ) ;
#25395=EDGE_CURVE ( 'NONE', #8379, #1305, #17852, .T. ) ;
#25397=CARTESIAN_POINT ( 'NONE',  ( 4.000000000000003553, 27.73750000000000071, 6.690598923241489970 ) ) ;
#25401=CARTESIAN_POINT ( 'NONE',  ( 3.469446951953614189E-15, 40.00000000000000000, 8.999999999999992895 ) ) ;
#25413=CARTESIAN_POINT ( 'NONE',  ( 3.834746474454188013E-15, 25.95624999877096428, 4.999999999999992006 ) ) ;
#25415=CARTESIAN_POINT ( 'NONE',  ( 3.756430356250004099, 28.89062499938548356, 6.831223922626973533 ) ) ;
#25425=CARTESIAN_POINT ( 'NONE',  ( -3.756430356249995661, 25.77812499938548640, 6.831223922626973533 ) ) ;
#25453=CARTESIAN_POINT ( 'NONE',  ( 3.756430356250003655, 26.60312499938548569, 8.999999999999992895 ) ) ;
#25462=AXIS2_PLACEMENT_3D ( 'NONE', #16695, #14600, #2701 ) ;
#25472=EDGE_CURVE ( 'NONE', #16189, #8379, #17818, .T. ) ;
#25476=CARTESIAN_POINT ( 'NONE',  ( 1.071796769724494558, 25.93615380933863435, 4.999999999999992895 ) ) ;
#25482=CARTESIAN_POINT ( 'NONE',  ( -3.756430356249997882, 27.31562499938548427, 11.16877607737301226 ) ) ;
#25489=DIRECTION ( 'NONE',  ( -0.000000000000000000, -1.000000000000000000, -0.000000000000000000 ) ) ;
#25516=ADVANCED_FACE ( 'NONE', ( #17318 ), #9716, .T. ) ;
#25533=CARTESIAN_POINT ( 'NONE',  ( -3.137519842735244810E-15, 26.91249999999999787, 4.999999999999991118 ) ) ;
#25536=CARTESIAN_POINT ( 'NONE',  ( -1.999999999999998224, 26.20000000000000284, 12.46410161513774639 ) ) ;
#25547=CARTESIAN_POINT ( 'NONE',  ( 2.000000000000000888, 25.82499999999999929, 12.46410161513774817 ) ) ;
#25558=CARTESIAN_POINT ( 'NONE',  ( 3.756430356250004099, 27.54062499938548569, 6.831223922626973533 ) ) ;
#25580=CARTESIAN_POINT ( 'NONE',  ( 1.859271017917182139E-15, 29.33124999877096428, 12.99999999999999289 ) ) ;
#25586=CARTESIAN_POINT ( 'NONE',  ( 4.000000000000003553, 25.88124999877096499, 6.690598923241489970 ) ) ;
#25591=CARTESIAN_POINT ( 'NONE',  ( -1.878215178124998497, 29.15312499938548640, 12.25316411605951927 ) ) ;
#25595=LINE ( 'NONE', #25844, #6706 ) ;
#25599=AXIS2_PLACEMENT_3D ( 'NONE', #1481, #9835, #9452 ) ;
#25615=CARTESIAN_POINT ( 'NONE',  ( 3.735045420075836212E-15, 27.16562499938548569, 4.662447845253954171 ) ) ;
#25618=COLOUR_RGB ( '',0.8941176470588234615, 0.8941176470588234615, 0.8941176470588234615 ) ;
#25623=CYLINDRICAL_SURFACE ( 'NONE', #20878, 4.000000000000000000 ) ;
#25634=DIRECTION ( 'NONE',  ( 0.000000000000000000, 0.000000000000000000, -1.000000000000000000 ) ) ;
#25647=( BOUNDED_CURVE ( )  B_SPLINE_CURVE ( 2, ( #24676, #8862, #6621, #6498, #24811, #14483, #10799, #10937, #10547 ),
 .UNSPECIFIED., .F., .T. ) 
 B_SPLINE_CURVE_WITH_KNOTS ( ( 3, 2, 2, 2, 3 ),
 ( 0.5750000000000000666, 0.5833333333333333703, 0.5999999999999999778, 0.6166666666666666963, 0.6250000000000000000 ),
 .UNSPECIFIED. ) 
 CURVE ( )  GEOMETRIC_REPRESENTATION_ITEM ( )  RATIONAL_B_SPLINE_CURVE ( ( 0.9330127018922194093, 0.9330127018922198534, 1.000000000000000000, 0.8660254037844387076, 1.000000000000000000, 0.8660254037844387076, 1.000000000000000000, 0.9330127018922194093, 0.9330127018922194093 ) ) 
 REPRESENTATION_ITEM ( '' )  );
#25666=CARTESIAN_POINT ( 'NONE',  ( 4.000000000000001776, 27.66249999999999787, 11.30940107675849760 ) ) ;
#25682=CARTESIAN_POINT ( 'NONE',  ( -1.999999999999995781, 25.99374999877096926, 5.535898384862237620 ) ) ;
#25684=CARTESIAN_POINT ( 'NONE',  ( -1.878215178124995832, 29.45312499938548356, 5.746835883940462963 ) ) ;
#25695=CARTESIAN_POINT ( 'NONE',  ( 3.469446951953614189E-15, 40.00000000000000000, 8.999999999999992895 ) ) ;
#25699=CARTESIAN_POINT ( 'NONE',  ( -1.071796769724481901, 27.56740381056766864, 12.99999999999999645 ) ) ;
#25711=CARTESIAN_POINT ( 'NONE',  ( -3.999999999999996447, 27.86874999877096570, 8.999999999999992895 ) ) ;
#25714=CARTESIAN_POINT ( 'NONE',  ( -1.878215178124995832, 28.10312499938548569, 5.746835883940462963 ) ) ;
#25719=ORIENTED_EDGE ( 'NONE', *, *, #3811, .T. ) ;
#25728=CARTESIAN_POINT ( 'NONE',  ( 4.000000000000003553, 29.69687499938548569, 8.999999999999992895 ) ) ;
#25733=EDGE_LOOP ( 'NONE', ( #15723, #8382, #7318, #21373, #7372, #9737, #7816, #222, #19135, #12710, #10205, #4000, #9946, #4974, #11431, #12035, #6996, #1085, #25748, #1472, #19914, #3696, #2493, #12358 ) ) ;
#25736=CARTESIAN_POINT ( 'NONE',  ( 1.878215178125004048, 28.47812499938548569, 5.746835883940462963 ) ) ;
#25737=CARTESIAN_POINT ( 'NONE',  ( -1.071796769724488563, 29.76115380933863364, 12.99999999999999289 ) ) ;
#25746=ORIENTED_EDGE ( 'NONE', *, *, #7935, .T. ) ;
#25748=ORIENTED_EDGE ( 'NONE', *, *, #5402, .F. ) ;
#25752=CARTESIAN_POINT ( 'NONE',  ( 8.831537335106614961E-15, 26.63124999877096855, 12.99999999999999112 ) ) ;
#25760=DIRECTION ( 'NONE',  ( 0.000000000000000000, 1.000000000000000000, 0.000000000000000000 ) ) ;
#25782=CARTESIAN_POINT ( 'NONE',  ( -3.999999999999996447, 29.27500000000000213, 8.999999999999992895 ) ) ;
#25788=( BOUNDED_CURVE ( )  B_SPLINE_CURVE ( 2, ( #14848, #3073, #15111, #21236, #13014, #16941, #23085, #13148, #6986 ),
 .UNSPECIFIED., .F., .F. ) 
 B_SPLINE_CURVE_WITH_KNOTS ( ( 3, 2, 2, 2, 3 ),
 ( 0.4250000000000000444, 0.4333333333333333481, 0.4500000000000000111, 0.4666666666666666741, 0.4750000000000000333 ),
 .UNSPECIFIED. ) 
 CURVE ( )  GEOMETRIC_REPRESENTATION_ITEM ( )  RATIONAL_B_SPLINE_CURVE ( ( 0.9330127018922194093, 0.9330127018922196314, 1.000000000000000000, 0.8660254037844387076, 1.000000000000000000, 0.8660254037844387076, 1.000000000000000000, 0.9330127018922191873, 0.9330127018922194093 ) ) 
 REPRESENTATION_ITEM ( '' )  );
#25797=CARTESIAN_POINT ( 'NONE',  ( -3.999999999999997335, 29.31250000000000000, 11.30940107675849404 ) ) ;
#25809=ORIENTED_EDGE ( 'NONE', *, *, #7384, .T. ) ;
#25830=CARTESIAN_POINT ( 'NONE',  ( 4.000000000000003553, 29.44374999877096855, 8.999999999999992895 ) ) ;
#25837=CARTESIAN_POINT ( 'NONE',  ( 2.000000000000003997, 28.61874999877096926, 5.535898384862238508 ) ) ;
#25841=CARTESIAN_POINT ( 'NONE',  ( -3.756430356249996994, 27.27812499938548640, 8.999999999999992895 ) ) ;
#25844=CARTESIAN_POINT ( 'NONE',  ( 4.143002691484658293E-15, 46.00000000000000000, 14.49999999999999289 ) ) ;
#25864=CARTESIAN_POINT ( 'NONE',  ( 3.735045420075836212E-15, 26.71562499938548640, 4.662447845253954171 ) ) ;
#25867=CARTESIAN_POINT ( 'NONE',  ( -3.999999999999996447, 29.66874999877096997, 8.999999999999992895 ) ) ;
#25922=COLOUR_RGB('Off White',0.89,0.88,0.83);
#25923=FILL_AREA_STYLE_COLOUR('',#25922);
#25924=FILL_AREA_STYLE('',(#25923));
#25925=SURFACE_STYLE_FILL_AREA(#25924);
#25926=SURFACE_SIDE_STYLE('',(#25925));
#25927=SURFACE_STYLE_USAGE(.BOTH.,#25926);
#25928=PRESENTATION_STYLE_ASSIGNMENT((#25927));
ENDSEC;
END-ISO-10303-21;
